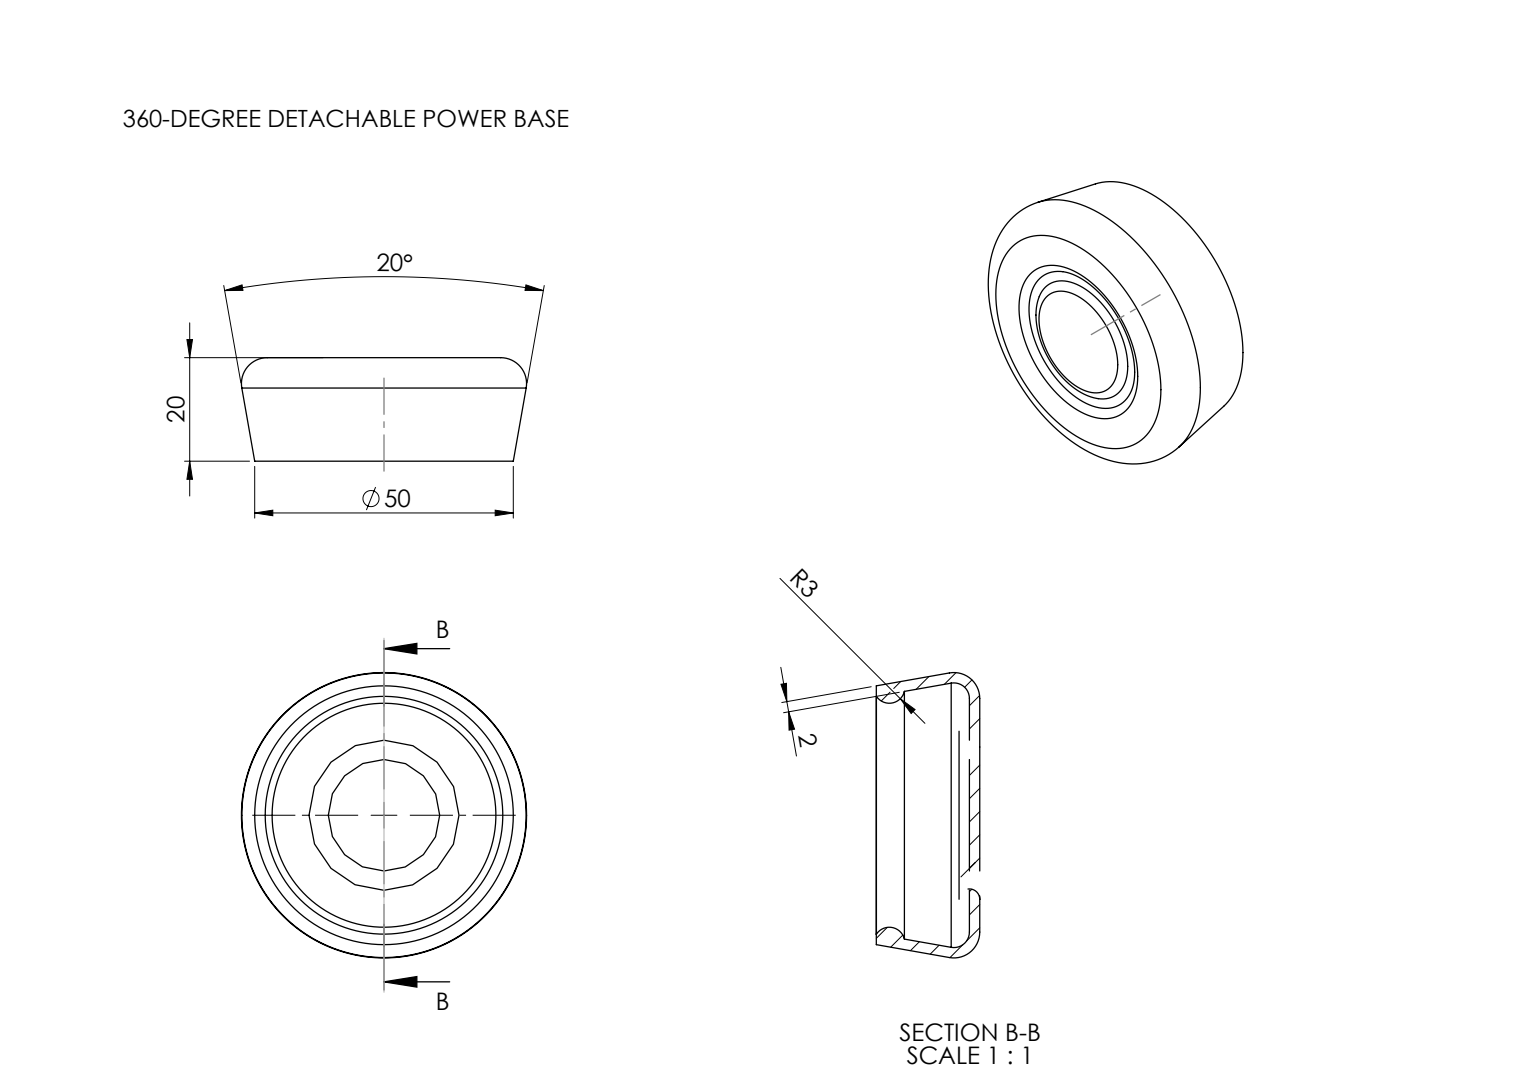
ISO-10303-21;
HEADER;
FILE_DESCRIPTION (('STEP AP214'),
    '1' );
FILE_NAME ('360-Degree Detachable Power Base.step',
    '2026-10-08T15:02:10',
    ( '' ),
    ( '' ),
    'SwSTEP 2.0',
    'SolidWorks 2026',
    '' );
FILE_SCHEMA (( 'AUTOMOTIVE_DESIGN' ));
ENDSEC;

DATA;
#9=ORIENTED_EDGE ( 'NONE', *, *, #11620, .F. ) ;
#88=AXIS2_PLACEMENT_3D ( 'NONE', #22054, #11930, #10248 ) ;
#91=AXIS2_PLACEMENT_3D ( 'NONE', #18121, #12939, #8104 ) ;
#101=CARTESIAN_POINT ( 'NONE',  ( -0.6349943332661909245, -10.75744069813302417, 92.00000000000001421 ) ) ;
#115=CARTESIAN_POINT ( 'NONE',  ( 23.92685091328690916, 0.000000000000000000, 80.43141006107198621 ) ) ;
#133=CIRCLE ( 'NONE', #6226, 27.49181041625929112 ) ;
#192=CIRCLE ( 'NONE', #12763, 23.92685091328691271 ) ;
#217=CARTESIAN_POINT ( 'NONE',  ( 0.000000000000000000, 0.000000000000000000, 75.00000000000000000 ) ) ;
#237=VERTEX_POINT ( 'NONE', #7603 ) ;
#250=EDGE_CURVE ( 'NONE', #10146, #1916, #14804, .T. ) ;
#282=SURFACE_STYLE_FILL_AREA ( #6812 ) ;
#298=ORIENTED_EDGE ( 'NONE', *, *, #2080, .T. ) ;
#311=DIRECTION ( 'NONE',  ( -0.1736481776669307198, 2.126576849575776229E-17, 0.9848077530122080203 ) ) ;
#428=ORIENTED_EDGE ( 'NONE', *, *, #5250, .F. ) ;
#434=DIRECTION ( 'NONE',  ( 0.000000000000000000, -1.000000000000000000, 0.000000000000000000 ) ) ;
#489=CARTESIAN_POINT ( 'NONE',  ( 0.000000000000000000, 0.000000000000000000, 75.01817430661621700 ) ) ;
#497=VERTEX_POINT ( 'NONE', #16816 ) ;
#506=CARTESIAN_POINT ( 'NONE',  ( 22.56777165119825668, 0.000000000000000000, 90.00000000000000000 ) ) ;
#515=LINE ( 'NONE', #19075, #11094 ) ;
#527=CARTESIAN_POINT ( 'NONE',  ( 0.000000000000000000, 0.000000000000000000, 93.00000000000000000 ) ) ;
#552=CARTESIAN_POINT ( 'NONE',  ( -10.76794919243112325, -2.704190363445815236E-15, 92.00000000000000000 ) ) ;
#572=LINE ( 'NONE', #18015, #14095 ) ;
#626=CARTESIAN_POINT ( 'NONE',  ( 0.000000000000000000, 0.000000000000000000, 94.00000000000000000 ) ) ;
#627=EDGE_CURVE ( 'NONE', #17378, #2791, #3286, .T. ) ;
#680=CARTESIAN_POINT ( 'NONE',  ( -1.701984465643862965, -14.42982486328545377, 93.00000000000000000 ) ) ;
#751=ADVANCED_FACE ( 'NONE', ( #21864, #18061 ), #2957, .F. ) ;
#779=CARTESIAN_POINT ( 'NONE',  ( 0.4310340159982882779, 14.49716617963122189, 93.00000000000001421 ) ) ;
#825=DIRECTION ( 'NONE',  ( 1.000000000000000000, 0.000000000000000000, 0.000000000000000000 ) ) ;
#840=DIRECTION ( 'NONE',  ( 1.000000000000000000, 0.000000000000000000, 0.000000000000000000 ) ) ;
#846=VERTEX_POINT ( 'NONE', #22098 ) ;
#895=CARTESIAN_POINT ( 'NONE',  ( -4.825543794723682112, 13.95218839875094829, 93.00000000000001421 ) ) ;
#912=CARTESIAN_POINT ( 'NONE',  ( 0.000000000000000000, 0.000000000000000000, 93.00000000000000000 ) ) ;
#930=VERTEX_POINT ( 'NONE', #1922 ) ;
#945=VERTEX_POINT ( 'NONE', #13560 ) ;
#980=CARTESIAN_POINT ( 'NONE',  ( 0.000000000000000000, 0.000000000000000000, 95.00000000000000000 ) ) ;
#1005=ORIENTED_EDGE ( 'NONE', *, *, #4139, .T. ) ;
#1007=CARTESIAN_POINT ( 'NONE',  ( 6.453512288987237611, 13.27786176931083695, 93.00000000000000000 ) ) ;
#1012=CARTESIAN_POINT ( 'NONE',  ( 13.08434944240164022, -7.394545551606342748, 92.99999999999998579 ) ) ;
#1024=DIRECTION ( 'NONE',  ( 1.000000000000000000, 0.000000000000000000, 0.000000000000000000 ) ) ;
#1027=EDGE_CURVE ( 'NONE', #7787, #237, #6904, .T. ) ;
#1132=DIRECTION ( 'NONE',  ( 1.000000000000000000, 0.000000000000000000, 0.000000000000000000 ) ) ;
#1155=AXIS2_PLACEMENT_3D ( 'NONE', #10454, #3681, #5262 ) ;
#1180=ORIENTED_EDGE ( 'NONE', *, *, #8054, .T. ) ;
#1188=AXIS2_PLACEMENT_3D ( 'NONE', #7802, #21501, #4395 ) ;
#1209=CONICAL_SURFACE ( 'NONE', #1910, 23.03038449397558196, 0.1745329251994333364 ) ;
#1245=CARTESIAN_POINT ( 'NONE',  ( 10.76794919243112325, 1.318693451189210089E-15, 93.00000000000000000 ) ) ;
#1307=VECTOR ( 'NONE', #17008, 1000.000000000000000 ) ;
#1311=ADVANCED_FACE ( 'NONE', ( #17464 ), #8333, .T. ) ;
#1322=FILL_AREA_STYLE_COLOUR ( '', #5562 ) ;
#1341=CARTESIAN_POINT ( 'NONE',  ( -14.49943138577569535, 0.2467007162552621036, 93.00000000000002842 ) ) ;
#1423=EDGE_CURVE ( 'NONE', #10960, #18642, #18111, .T. ) ;
#1436=EDGE_CURVE ( 'NONE', #1916, #930, #572, .T. ) ;
#1451=CARTESIAN_POINT ( 'NONE',  ( 10.76794919243112325, 0.000000000000000000, 92.00000000000000000 ) ) ;
#1464=CARTESIAN_POINT ( 'NONE',  ( 0.000000000000000000, 0.000000000000000000, 89.47905546699919910 ) ) ;
#1514=ORIENTED_EDGE ( 'NONE', *, *, #6789, .T. ) ;
#1566=CARTESIAN_POINT ( 'NONE',  ( 1.509788170712047295, -10.75822951548915007, 92.00000000000001421 ) ) ;
#1680=CARTESIAN_POINT ( 'NONE',  ( -7.838405800256100342, -7.387516090585425133, 92.00000000000000000 ) ) ;
#1686=ADVANCED_FACE ( 'NONE', ( #14531, #18010 ), #13270, .T. ) ;
#1755=CIRCLE ( 'NONE', #9316, 22.56777165119825668 ) ;
#1758=ORIENTED_EDGE ( 'NONE', *, *, #16835, .F. ) ;
#1790=CARTESIAN_POINT ( 'NONE',  ( 0.04718088033475073551, 10.76825293233556025, 91.99999999999998579 ) ) ;
#1832=EDGE_CURVE ( 'NONE', #18642, #10960, #2554, .T. ) ;
#1898=AXIS2_PLACEMENT_3D ( 'NONE', #489, #17488, #19159 ) ;
#1910=AXIS2_PLACEMENT_3D ( 'NONE', #9554, #18324, #18550 ) ;
#1916=VERTEX_POINT ( 'NONE', #20680 ) ;
#1922=CARTESIAN_POINT ( 'NONE',  ( -22.97235139684061878, 2.813301660702908866E-15, 75.01817430661621700 ) ) ;
#1975=CARTESIAN_POINT ( 'NONE',  ( -16.23205080756887853, 1.987852906508643644E-15, 93.00000000000000000 ) ) ;
#1976=EDGE_LOOP ( 'NONE', ( #12539, #12676 ) ) ;
#1979=DIRECTION ( 'NONE',  ( 1.000000000000000000, 0.000000000000000000, 0.000000000000000000 ) ) ;
#1982=CIRCLE ( 'NONE', #17819, 3.000000000000030198 ) ;
#1991=CARTESIAN_POINT ( 'NONE',  ( 0.000000000000000000, 0.000000000000000000, 89.47905546699919910 ) ) ;
#2000=ORIENTED_EDGE ( 'NONE', *, *, #16135, .T. ) ;
#2018=DIRECTION ( 'NONE',  ( 1.000000000000000000, 0.000000000000000000, 0.000000000000000000 ) ) ;
#2028=CIRCLE ( 'NONE', #16770, 23.92685091328691271 ) ;
#2068=ORIENTED_EDGE ( 'NONE', *, *, #1832, .F. ) ;
#2079=ORIENTED_EDGE ( 'NONE', *, *, #3880, .F. ) ;
#2080=EDGE_CURVE ( 'NONE', #10588, #846, #3065, .T. ) ;
#2089=DIRECTION ( 'NONE',  ( 1.000000000000000000, 0.000000000000000000, 0.000000000000000000 ) ) ;
#2124=CARTESIAN_POINT ( 'NONE',  ( -10.75744069813302417, 0.6349943332661998063, 92.00000000000000000 ) ) ;
#2128=DIRECTION ( 'NONE',  ( 0.000000000000000000, 0.000000000000000000, 1.000000000000000000 ) ) ;
#2143=CARTESIAN_POINT ( 'NONE',  ( 0.000000000000000000, 0.000000000000000000, 93.00000000000000000 ) ) ;
#2163=DIRECTION ( 'NONE',  ( 0.000000000000000000, 0.000000000000000000, 1.000000000000000000 ) ) ;
#2175=DIRECTION ( 'NONE',  ( 1.000000000000000000, 0.000000000000000000, 0.000000000000000000 ) ) ;
#2192=ADVANCED_FACE ( 'NONE', ( #8994 ), #7283, .T. ) ;
#2236=DIRECTION ( 'NONE',  ( 0.000000000000000000, 0.000000000000000000, -1.000000000000000000 ) ) ;
#2274=TOROIDAL_SURFACE ( 'NONE', #3700, 10.76794919243112325, 2.000000000000000000 ) ;
#2295=AXIS2_PLACEMENT_3D ( 'NONE', #9527, #19416, #4437 ) ;
#2358=EDGE_CURVE ( 'NONE', #20525, #20136, #5458, .T. ) ;
#2364=CIRCLE ( 'NONE', #7779, 25.52219491023488018 ) ;
#2425=DIRECTION ( 'NONE',  ( 0.000000000000000000, 0.000000000000000000, 1.000000000000000000 ) ) ;
#2452=AXIS2_PLACEMENT_3D ( 'NONE', #1975, #17738, #14032 ) ;
#2465=CARTESIAN_POINT ( 'NONE',  ( 10.60004861036625812, 9.899508790423018567, 93.00000000000001421 ) ) ;
#2554=B_SPLINE_CURVE_WITH_KNOTS ( 'NONE', 3,
 ( #16647, #17902, #11364, #9458, #4366, #21473, #2465, #9348, #9676, #16208, #1007, #13049, #19897, #20008, #779, #21811, #16319, #4485, #11470, #895, #5957, #18233, #12834, #7771, #16535, #7989, #6289, #13163, #4594, #18677, #3131, #10122, #6511, #1341, #15418, #15085, #16763 ),
 .UNSPECIFIED., .F., .F.,
 ( 4, 1, 1, 1, 1, 2, 2, 1, 1, 1, 1, 1, 2, 2, 1, 1, 1, 1, 1, 2, 2, 1, 1, 1, 1, 1, 2, 4 ),
 ( 0.000000000000000000, 0.06249999999999955591, 0.09374999999999931999, 0.1093749999999992090, 0.1171874999999991673, 0.1210937499999991673, 0.1249999999999991673, 0.1874999999999990008, 0.2187499999999988898, 0.2343749999999988343, 0.2421874999999988065, 0.2460937499999987788, 0.2480468749999987510, 0.2499999999999987788, 0.3124999999999985012, 0.3437499999999983902, 0.3593749999999983347, 0.3671874999999983347, 0.3710937499999982792, 0.3730468749999982792, 0.3749999999999982792, 0.4374999999999991118, 0.4687499999999995559, 0.4843749999999997780, 0.4921874999999998890, 0.4960937499999998890, 0.4980468749999999445, 0.5000000000000000000 ),
 .UNSPECIFIED. ) ;
#2582=AXIS2_PLACEMENT_3D ( 'NONE', #11523, #4313, #9844 ) ;
#2633=EDGE_CURVE ( 'NONE', #15441, #11225, #10382, .T. ) ;
#2661=VERTEX_POINT ( 'NONE', #13953 ) ;
#2665=AXIS2_PLACEMENT_3D ( 'NONE', #9411, #17753, #7839 ) ;
#2668=UNCERTAINTY_MEASURE_WITH_UNIT (LENGTH_MEASURE( 1.000000000000000082E-05 ), #5436, 'distance_accuracy_value', 'NONE');
#2693=CARTESIAN_POINT ( 'NONE',  ( -14.49031849020019003, -2.025093002184656488, 93.00000000000000000 ) ) ;
#2705=CARTESIAN_POINT ( 'NONE',  ( 0.000000000000000000, 0.000000000000000000, 93.00000000000000000 ) ) ;
#2707=DIRECTION ( 'NONE',  ( 1.000000000000000000, 0.000000000000000000, 0.000000000000000000 ) ) ;
#2791=VERTEX_POINT ( 'NONE', #12914 ) ;
#2814=DIRECTION ( 'NONE',  ( 0.000000000000000000, 0.000000000000000000, 1.000000000000000000 ) ) ;
#2837=CARTESIAN_POINT ( 'NONE',  ( -16.23205080756887853, 1.987852906508643644E-15, 95.00000000000000000 ) ) ;
#2853=VERTEX_POINT ( 'NONE', #17880 ) ;
#2888=AXIS2_PLACEMENT_3D ( 'NONE', #4214, #14918, #840 ) ;
#2957=PLANE ( 'NONE',  #2582 ) ;
#3012=ORIENTED_EDGE ( 'NONE', *, *, #250, .T. ) ;
#3015=CARTESIAN_POINT ( 'NONE',  ( 7.354678144329572120, -7.869443266638024070, 92.00000000000000000 ) ) ;
#3026=CARTESIAN_POINT ( 'NONE',  ( 8.476473295508071715, 6.680697330908218490, 92.00000000000002842 ) ) ;
#3065=B_SPLINE_CURVE_WITH_KNOTS ( 'NONE', 3,
 ( #13724, #12032, #22158, #15194, #11810, #4820, #1680, #9899, #6856, #18784, #6971, #16987, #20338, #17208, #101, #15518, #8324, #13843, #11918, #1566, #11697, #8554, #6747, #11577, #3015, #4934, #18566, #8441, #10011, #1451 ),
 .UNSPECIFIED., .F., .F.,
 ( 4, 1, 1, 1, 1, 1, 2, 2, 1, 1, 1, 1, 1, 2, 2, 1, 1, 1, 1, 2, 2, 4 ),
 ( 0.5000000000000000000, 0.5625000000000000000, 0.5937500000000000000, 0.6093750000000001110, 0.6171875000000001110, 0.6210937500000001110, 0.6230468750000001110, 0.6250000000000001110, 0.6875000000000002220, 0.7187500000000003331, 0.7343750000000003331, 0.7421875000000003331, 0.7460937500000003331, 0.7480468750000003331, 0.7500000000000004441, 0.8125000000000004441, 0.8437500000000004441, 0.8593750000000005551, 0.8671875000000005551, 0.8710937500000006661, 0.8750000000000006661, 1.000000000000000000 ),
 .UNSPECIFIED. ) ;
#3073=EDGE_CURVE ( 'NONE', #2853, #20136, #1755, .T. ) ;
#3111=( LENGTH_UNIT ( ) NAMED_UNIT ( * ) SI_UNIT ( .MILLI., .METRE. ) );
#3131=CARTESIAN_POINT ( 'NONE',  ( -14.42982486328545200, 1.701984465643896272, 93.00000000000001421 ) ) ;
#3140=CARTESIAN_POINT ( 'NONE',  ( 0.3188271712753663611, 10.76635261883074257, 92.00000000000001421 ) ) ;
#3142=FACE_BOUND ( 'NONE', #22130, .T. ) ;
#3168=AXIS2_PLACEMENT_3D ( 'NONE', #13351, #18422, #4789 ) ;
#3286=CIRCLE ( 'NONE', #10846, 10.76794919243112325 ) ;
#3316=AXIS2_PLACEMENT_3D ( 'NONE', #1464, #11824, #18690 ) ;
#3322=ORIENTED_EDGE ( 'NONE', *, *, #12216, .F. ) ;
#3334=DIRECTION ( 'NONE',  ( 1.224646799147353207E-16, 1.000000000000000000, -0.000000000000000000 ) ) ;
#3348=ORIENTED_EDGE ( 'NONE', *, *, #13732, .T. ) ;
#3361=EDGE_CURVE ( 'NONE', #6741, #945, #20046, .T. ) ;
#3465=ORIENTED_EDGE ( 'NONE', *, *, #250, .F. ) ;
#3530=SURFACE_STYLE_USAGE ( .BOTH. , #18954 ) ;
#3630=EDGE_CURVE ( 'NONE', #4483, #16572, #12535, .T. ) ;
#3633=ORIENTED_EDGE ( 'NONE', *, *, #20686, .F. ) ;
#3681=DIRECTION ( 'NONE',  ( -0.000000000000000000, -0.000000000000000000, 1.000000000000000000 ) ) ;
#3688=AXIS2_PLACEMENT_3D ( 'NONE', #12548, #7157, #12442 ) ;
#3700=AXIS2_PLACEMENT_3D ( 'NONE', #20546, #10329, #10549 ) ;
#3795=CIRCLE ( 'NONE', #21027, 2.000000000000001776 ) ;
#3806=B_SPLINE_CURVE_WITH_KNOTS ( 'NONE', 3,
 ( #6756, #8666, #5160, #4944, #3026, #8563, #18578, #20235, #10023, #20123, #4831, #11928, #15427, #6865, #3140, #11590, #15529, #1790, #18462, #9913, #16776, #8224, #6522, #13392, #8335, #11820, #12378, #3809, #17662, #19008, #17325, #2124, #17779, #10462, #8895, #13961, #552 ),
 .UNSPECIFIED., .F., .F.,
 ( 4, 1, 1, 1, 1, 2, 2, 1, 1, 1, 1, 1, 2, 2, 1, 1, 1, 1, 1, 2, 2, 1, 1, 1, 1, 1, 2, 4 ),
 ( 0.000000000000000000, 0.06250000000000048572, 0.09375000000000069389, 0.1093750000000008049, 0.1171875000000008604, 0.1210937500000009159, 0.1250000000000009714, 0.1875000000000012212, 0.2187500000000013600, 0.2343750000000014433, 0.2421875000000014710, 0.2460937500000014710, 0.2480468750000014710, 0.2500000000000014988, 0.3125000000000016653, 0.3437500000000017208, 0.3593750000000017764, 0.3671875000000017764, 0.3710937500000017764, 0.3730468750000017208, 0.3750000000000016653, 0.4375000000000008882, 0.4687500000000004996, 0.4843750000000002776, 0.4921875000000001665, 0.4960937500000000555, 0.4980468750000000555, 0.5000000000000000000 ),
 .UNSPECIFIED. ) ;
#3809=CARTESIAN_POINT ( 'NONE',  ( -8.674798497629360838, 6.539635590297948831, 91.99999999999997158 ) ) ;
#3822=AXIS2_PLACEMENT_3D ( 'NONE', #18252, #2814, #13071 ) ;
#3880=EDGE_CURVE ( 'NONE', #10146, #945, #515, .T. ) ;
#3886=SHAPE_REPRESENTATION_RELATIONSHIP ( 'NONE' , 'NONE' ,  #8462, #21175 ) ;
#3889=ORIENTED_EDGE ( 'NONE', *, *, #8253, .F. ) ;
#3912=ORIENTED_EDGE ( 'NONE', *, *, #3073, .F. ) ;
#3931=ORIENTED_EDGE ( 'NONE', *, *, #17519, .T. ) ;
#3969=ORIENTED_EDGE ( 'NONE', *, *, #8054, .F. ) ;
#4000=FACE_OUTER_BOUND ( 'NONE', #15773, .T. ) ;
#4003=EDGE_CURVE ( 'NONE', #12254, #20879, #20779, .T. ) ;
#4023=UNCERTAINTY_MEASURE_WITH_UNIT (LENGTH_MEASURE( 1.000000000000000082E-05 ), #4912, 'distance_accuracy_value', 'NONE');
#4042=TOROIDAL_SURFACE ( 'NONE', #8734, 22.56777165119825668, 5.000000000000000000 ) ;
#4049=CARTESIAN_POINT ( 'NONE',  ( -0.06328415631827169485, -14.50030254718124390, 92.99999999999998579 ) ) ;
#4084=FACE_OUTER_BOUND ( 'NONE', #17806, .T. ) ;
#4093=TOROIDAL_SURFACE ( 'NONE', #2665, 24.63401512838761320, 3.000000000000035083 ) ;
#4139=EDGE_CURVE ( 'NONE', #21337, #16572, #10736, .T. ) ;
#4160=CARTESIAN_POINT ( 'NONE',  ( 14.50000000000000000, 0.000000000000000000, 93.00000000000000000 ) ) ;
#4169=ADVANCED_FACE ( 'NONE', ( #20868 ), #14696, .T. ) ;
#4170=EDGE_LOOP ( 'NONE', ( #21486, #15699, #13268, #3912 ) ) ;
#4194=DIRECTION ( 'NONE',  ( -1.000000000000000000, -1.224646799147353454E-16, 0.000000000000000000 ) ) ;
#4214=CARTESIAN_POINT ( 'NONE',  ( 0.000000000000000000, 0.000000000000000000, 75.34729635533385306 ) ) ;
#4269=CARTESIAN_POINT ( 'NONE',  ( -14.50000000000000000, 1.775737858763662015E-15, 93.00000000000000000 ) ) ;
#4313=DIRECTION ( 'NONE',  ( 0.000000000000000000, 0.000000000000000000, 1.000000000000000000 ) ) ;
#4357=DIRECTION ( 'NONE',  ( -0.000000000000000000, -0.000000000000000000, -1.000000000000000000 ) ) ;
#4366=CARTESIAN_POINT ( 'NONE',  ( 11.41432417523484055, 8.992600385930652251, 93.00000000000000000 ) ) ;
#4372=CARTESIAN_POINT ( 'NONE',  ( -10.42709000561872834, -10.07820250684338603, 93.00000000000001421 ) ) ;
#4380=ORIENTED_EDGE ( 'NONE', *, *, #12449, .F. ) ;
#4395=DIRECTION ( 'NONE',  ( 1.000000000000000000, 0.000000000000000000, 0.000000000000000000 ) ) ;
#4437=DIRECTION ( 'NONE',  ( 1.000000000000000000, 0.000000000000000000, 0.000000000000000000 ) ) ;
#4445=DIRECTION ( 'NONE',  ( 0.000000000000000000, -1.000000000000000000, 0.000000000000000000 ) ) ;
#4483=VERTEX_POINT ( 'NONE', #18176 ) ;
#4485=CARTESIAN_POINT ( 'NONE',  ( 0.06328415631827062626, 14.50030254718124212, 92.99999999999997158 ) ) ;
#4579=CARTESIAN_POINT ( 'NONE',  ( 0.000000000000000000, 0.000000000000000000, 89.13175911166534604 ) ) ;
#4594=CARTESIAN_POINT ( 'NONE',  ( -13.27786176931083162, 6.453512288987280243, 92.99999999999998579 ) ) ;
#4657=ORIENTED_EDGE ( 'NONE', *, *, #13403, .T. ) ;
#4776=AXIS2_PLACEMENT_3D ( 'NONE', #12920, #16411, #9331 ) ;
#4789=DIRECTION ( 'NONE',  ( 1.000000000000000000, 0.000000000000000000, 0.000000000000000000 ) ) ;
#4790=ORIENTED_EDGE ( 'NONE', *, *, #20520, .F. ) ;
#4820=CARTESIAN_POINT ( 'NONE',  ( -8.055668064929562888, -7.157650466794454935, 91.99999999999997158 ) ) ;
#4831=CARTESIAN_POINT ( 'NONE',  ( 4.782033626261160464, 9.864562363145058299, 92.00000000000000000 ) ) ;
#4912=( LENGTH_UNIT ( ) NAMED_UNIT ( * ) SI_UNIT ( .MILLI., .METRE. ) );
#4934=CARTESIAN_POINT ( 'NONE',  ( 7.485089409085513346, -7.743278074783935594, 91.99999999999998579 ) ) ;
#4944=CARTESIAN_POINT ( 'NONE',  ( 9.223872243966841467, 5.696734612111038487, 92.00000000000001421 ) ) ;
#4951=DIRECTION ( 'NONE',  ( -0.000000000000000000, -0.000000000000000000, 1.000000000000000000 ) ) ;
#5042=ORIENTED_EDGE ( 'NONE', *, *, #13039, .F. ) ;
#5059=DIRECTION ( 'NONE',  ( 1.000000000000000000, 0.000000000000000000, 0.000000000000000000 ) ) ;
#5077=ORIENTED_EDGE ( 'NONE', *, *, #1027, .F. ) ;
#5101=EDGE_LOOP ( 'NONE', ( #14716, #20263, #18999, #19285 ) ) ;
#5132=CIRCLE ( 'NONE', #10175, 25.00000000000000000 ) ;
#5160=CARTESIAN_POINT ( 'NONE',  ( 10.37371678005726139, 3.577098705721246219, 91.99999999999998579 ) ) ;
#5216=ORIENTED_EDGE ( 'NONE', *, *, #21646, .F. ) ;
#5250=EDGE_CURVE ( 'NONE', #21337, #12667, #10141, .T. ) ;
#5262=DIRECTION ( 'NONE',  ( 1.000000000000000000, 0.000000000000000000, 0.000000000000000000 ) ) ;
#5317=AXIS2_PLACEMENT_3D ( 'NONE', #11889, #6371, #14944 ) ;
#5323=ORIENTED_EDGE ( 'NONE', *, *, #3630, .F. ) ;
#5332=DIRECTION ( 'NONE',  ( 0.000000000000000000, 0.000000000000000000, 1.000000000000000000 ) ) ;
#5387=ORIENTED_EDGE ( 'NONE', *, *, #10065, .T. ) ;
#5436=( LENGTH_UNIT ( ) NAMED_UNIT ( * ) SI_UNIT ( .MILLI., .METRE. ) );
#5443=CARTESIAN_POINT ( 'NONE',  ( 0.000000000000000000, 0.000000000000000000, 77.51594804401857175 ) ) ;
#5458=CIRCLE ( 'NONE', #12440, 5.000000000000004441 ) ;
#5465=VERTEX_POINT ( 'NONE', #15166 ) ;
#5494=AXIS2_PLACEMENT_3D ( 'NONE', #5443, #5670, #19502 ) ;
#5518=DIRECTION ( 'NONE',  ( -1.000000000000000000, 1.224646799147353454E-16, 0.000000000000000000 ) ) ;
#5562=COLOUR_RGB ( '', 0.40784314, 0.44705882, 0.49803922) ;
#5670=DIRECTION ( 'NONE',  ( -0.000000000000000000, -0.000000000000000000, 1.000000000000000000 ) ) ;
#5698=ADVANCED_FACE ( 'NONE', ( #21204 ), #5824, .F. ) ;
#5722=CARTESIAN_POINT ( 'NONE',  ( 0.000000000000000000, 0.000000000000000000, 93.00000000000000000 ) ) ;
#5736=CARTESIAN_POINT ( 'NONE',  ( -3.344898002356346378, -14.20274344593240912, 93.00000000000001421 ) ) ;
#5802=DIRECTION ( 'NONE',  ( 1.000000000000000000, 0.000000000000000000, 0.000000000000000000 ) ) ;
#5824=TOROIDAL_SURFACE ( 'NONE', #7991, 22.56777165119825668, 3.000000000000000000 ) ;
#5825=EDGE_CURVE ( 'NONE', #20879, #12254, #6862, .T. ) ;
#5830=CARTESIAN_POINT ( 'NONE',  ( 0.000000000000000000, 0.000000000000000000, 75.01817430661621700 ) ) ;
#5847=CARTESIAN_POINT ( 'NONE',  ( -0.2467007162552578292, -14.49943138577569357, 93.00000000000002842 ) ) ;
#5883=DIRECTION ( 'NONE',  ( -1.224646799147353207E-16, 1.000000000000000000, 0.000000000000000000 ) ) ;
#5902=DIRECTION ( 'NONE',  ( 0.000000000000000000, 0.000000000000000000, 1.000000000000000000 ) ) ;
#5939=ADVANCED_FACE ( 'NONE', ( #19305 ), #14769, .F. ) ;
#5942=LINE ( 'NONE', #13149, #19177 ) ;
#5944=VECTOR ( 'NONE', #311, 1000.000000000000000 ) ;
#5955=ORIENTED_EDGE ( 'NONE', *, *, #3361, .F. ) ;
#5957=CARTESIAN_POINT ( 'NONE',  ( -7.677656142228050484, 12.40805626191516353, 93.00000000000000000 ) ) ;
#5986=DIRECTION ( 'NONE',  ( 1.000000000000000000, 0.000000000000000000, -0.000000000000000000 ) ) ;
#6011=CARTESIAN_POINT ( 'NONE',  ( 0.000000000000000000, 0.000000000000000000, 95.00000000000000000 ) ) ;
#6020=ORIENTED_EDGE ( 'NONE', *, *, #18896, .F. ) ;
#6108=DIRECTION ( 'NONE',  ( 0.000000000000000000, 0.000000000000000000, 1.000000000000000000 ) ) ;
#6137=ORIENTED_EDGE ( 'NONE', *, *, #7781, .T. ) ;
#6179=CARTESIAN_POINT ( 'NONE',  ( 10.07835692657692128, -10.42743089613093233, 93.00000000000002842 ) ) ;
#6193=CARTESIAN_POINT ( 'NONE',  ( -23.92685091328690916, 2.930194138463273749E-15, 80.43141006107198621 ) ) ;
#6226=AXIS2_PLACEMENT_3D ( 'NONE', #4579, #6381, #11234 ) ;
#6230=ADVANCED_FACE ( 'NONE', ( #7830 ), #12616, .F. ) ;
#6233=DIRECTION ( 'NONE',  ( 1.000000000000000000, 0.000000000000000000, 0.000000000000000000 ) ) ;
#6267=CIRCLE ( 'NONE', #14209, 2.000000000000000000 ) ;
#6280=DIRECTION ( 'NONE',  ( -1.000000000000000000, 0.000000000000000000, 0.000000000000000000 ) ) ;
#6289=CARTESIAN_POINT ( 'NONE',  ( -10.20851360429410981, 10.29801091644274180, 92.99999999999998579 ) ) ;
#6298=CIRCLE ( 'NONE', #16361, 3.000000000000002665 ) ;
#6309=DIRECTION ( 'NONE',  ( 0.000000000000000000, 0.000000000000000000, 1.000000000000000000 ) ) ;
#6334=CARTESIAN_POINT ( 'NONE',  ( 0.000000000000000000, 0.000000000000000000, 75.00000000000000000 ) ) ;
#6371=DIRECTION ( 'NONE',  ( 0.000000000000000000, -1.000000000000000000, 0.000000000000000000 ) ) ;
#6381=DIRECTION ( 'NONE',  ( -0.000000000000000000, -0.000000000000000000, -1.000000000000000000 ) ) ;
#6397=ORIENTED_EDGE ( 'NONE', *, *, #3880, .T. ) ;
#6477=ORIENTED_EDGE ( 'NONE', *, *, #1436, .F. ) ;
#6511=CARTESIAN_POINT ( 'NONE',  ( -14.49716617963121834, 0.4310340159982911645, 92.99999999999997158 ) ) ;
#6522=CARTESIAN_POINT ( 'NONE',  ( -7.157650466794449606, 8.055668064929562888, 92.00000000000001421 ) ) ;
#6582=DIRECTION ( 'NONE',  ( -0.000000000000000000, -0.000000000000000000, 1.000000000000000000 ) ) ;
#6677=AXIS2_PLACEMENT_3D ( 'NONE', #18028, #16226, #2707 ) ;
#6741=VERTEX_POINT ( 'NONE', #16173 ) ;
#6747=CARTESIAN_POINT ( 'NONE',  ( 6.688043756404092655, -8.469031667849375111, 92.00000000000000000 ) ) ;
#6756=CARTESIAN_POINT ( 'NONE',  ( 10.76794919243112325, 0.000000000000000000, 92.00000000000000000 ) ) ;
#6789=EDGE_CURVE ( 'NONE', #497, #10628, #2364, .T. ) ;
#6812=FILL_AREA_STYLE ('',( #12099 ) ) ;
#6829=ORIENTED_EDGE ( 'NONE', *, *, #5250, .T. ) ;
#6856=CARTESIAN_POINT ( 'NONE',  ( -7.678935899902896267, -7.549707216296320134, 92.00000000000001421 ) ) ;
#6862=CIRCLE ( 'NONE', #7937, 12.50000000000000000 ) ;
#6865=CARTESIAN_POINT ( 'NONE',  ( 0.6349943332661940332, 10.75744069813302595, 92.00000000000002842 ) ) ;
#6878=ORIENTED_EDGE ( 'NONE', *, *, #14385, .F. ) ;
#6904=CIRCLE ( 'NONE', #19462, 3.000000000000033751 ) ;
#6923=PRESENTATION_STYLE_ASSIGNMENT (( #3530 ) ) ;
#6940=CARTESIAN_POINT ( 'NONE',  ( 0.000000000000000000, 0.000000000000000000, 94.00000000000000000 ) ) ;
#6971=CARTESIAN_POINT ( 'NONE',  ( -6.539635590297925738, -8.674798497629369720, 92.00000000000001421 ) ) ;
#7000=STYLED_ITEM ( 'NONE', ( #6923 ), #14295 ) ;
#7020=( GEOMETRIC_REPRESENTATION_CONTEXT ( 3 ) GLOBAL_UNCERTAINTY_ASSIGNED_CONTEXT ( ( #4023 ) ) GLOBAL_UNIT_ASSIGNED_CONTEXT ( ( #4912, #11897, #17080 ) ) REPRESENTATION_CONTEXT ( 'NONE', 'WORKASPACE' ) );
#7060=CARTESIAN_POINT ( 'NONE',  ( 0.000000000000000000, 0.000000000000000000, 90.00000000000000000 ) ) ;
#7067=DIRECTION ( 'NONE',  ( 1.000000000000000000, 0.000000000000000000, 0.000000000000000000 ) ) ;
#7071=AXIS2_PLACEMENT_3D ( 'NONE', #912, #6309, #1132 ) ;
#7086=DIRECTION ( 'NONE',  ( 1.000000000000000000, 0.000000000000000000, 0.000000000000000000 ) ) ;
#7107=EDGE_LOOP ( 'NONE', ( #20848, #8716 ) ) ;
#7157=DIRECTION ( 'NONE',  ( 0.000000000000000000, 0.000000000000000000, 1.000000000000000000 ) ) ;
#7192=ORIENTED_EDGE ( 'NONE', *, *, #3073, .T. ) ;
#7218=ORIENTED_EDGE ( 'NONE', *, *, #20925, .F. ) ;
#7259=ORIENTED_EDGE ( 'NONE', *, *, #627, .T. ) ;
#7272=ORIENTED_EDGE ( 'NONE', *, *, #21646, .T. ) ;
#7283=TOROIDAL_SURFACE ( 'NONE', #1155, 24.63401512838761320, 3.000000000000035083 ) ;
#7292=LINE ( 'NONE', #15734, #5944 ) ;
#7382=DIRECTION ( 'NONE',  ( 0.000000000000000000, 0.000000000000000000, -1.000000000000000000 ) ) ;
#7391=DIRECTION ( 'NONE',  ( 1.000000000000000000, 0.000000000000000000, 0.000000000000000000 ) ) ;
#7413=ORIENTED_EDGE ( 'NONE', *, *, #12216, .T. ) ;
#7448=CARTESIAN_POINT ( 'NONE',  ( 4.825543794723634150, -13.95218839875094119, 92.99999999999997158 ) ) ;
#7481=ORIENTED_EDGE ( 'NONE', *, *, #6789, .F. ) ;
#7496=EDGE_CURVE ( 'NONE', #14323, #2661, #14623, .T. ) ;
#7502=DIRECTION ( 'NONE',  ( 0.000000000000000000, 0.000000000000000000, 1.000000000000000000 ) ) ;
#7546=EDGE_CURVE ( 'NONE', #16572, #4483, #16413, .T. ) ;
#7554=CARTESIAN_POINT ( 'NONE',  ( -13.95218839875094119, -4.825543794723769153, 93.00000000000000000 ) ) ;
#7591=DIRECTION ( 'NONE',  ( 0.000000000000000000, 0.000000000000000000, -1.000000000000000000 ) ) ;
#7603=CARTESIAN_POINT ( 'NONE',  ( -21.63401512838757768, 2.649402737968526106E-15, 77.51594804401857175 ) ) ;
#7661=VECTOR ( 'NONE', #14357, 1000.000000000000000 ) ;
#7732=EDGE_CURVE ( 'NONE', #237, #930, #22164, .T. ) ;
#7771=CARTESIAN_POINT ( 'NONE',  ( -9.946257437971052440, 10.55583158923998077, 93.00000000000001421 ) ) ;
#7779=AXIS2_PLACEMENT_3D ( 'NONE', #1991, #12356, #5802 ) ;
#7781=EDGE_CURVE ( 'NONE', #2661, #14323, #7792, .T. ) ;
#7787=VERTEX_POINT ( 'NONE', #6193 ) ;
#7792=CIRCLE ( 'NONE', #14977, 22.56777165119825668 ) ;
#7802=CARTESIAN_POINT ( 'NONE',  ( 0.000000000000000000, 0.000000000000000000, 89.13175911166534604 ) ) ;
#7830=FACE_OUTER_BOUND ( 'NONE', #16877, .T. ) ;
#7839=DIRECTION ( 'NONE',  ( 1.000000000000000000, 0.000000000000000000, 0.000000000000000000 ) ) ;
#7855=DIRECTION ( 'NONE',  ( 0.000000000000000000, 0.000000000000000000, 1.000000000000000000 ) ) ;
#7873=CARTESIAN_POINT ( 'NONE',  ( 0.000000000000000000, 0.000000000000000000, 93.00000000000000000 ) ) ;
#7887=CARTESIAN_POINT ( 'NONE',  ( -10.84906991693323164, -9.635142796197690984, 93.00000000000001421 ) ) ;
#7937=AXIS2_PLACEMENT_3D ( 'NONE', #626, #10656, #2089 ) ;
#7962=ORIENTED_EDGE ( 'NONE', *, *, #5825, .T. ) ;
#7987=EDGE_LOOP ( 'NONE', ( #428, #1005, #5323, #17175 ) ) ;
#7989=CARTESIAN_POINT ( 'NONE',  ( -10.16585704662448641, 10.34058050218014557, 93.00000000000000000 ) ) ;
#7991=AXIS2_PLACEMENT_3D ( 'NONE', #7060, #7502, #1979 ) ;
#8043=AXIS2_PLACEMENT_3D ( 'NONE', #17298, #3334, #10216 ) ;
#8054=EDGE_CURVE ( 'NONE', #11225, #20525, #14054, .T. ) ;
#8104=DIRECTION ( 'NONE',  ( 1.000000000000000000, 0.000000000000000000, -0.000000000000000000 ) ) ;
#8192=CARTESIAN_POINT ( 'NONE',  ( 25.00000000000000000, 0.000000000000000000, 75.00000000000000000 ) ) ;
#8224=CARTESIAN_POINT ( 'NONE',  ( -6.688043756404080220, 8.469031667849378664, 92.00000000000001421 ) ) ;
#8244=CARTESIAN_POINT ( 'NONE',  ( 0.000000000000000000, 0.000000000000000000, 95.00000000000000000 ) ) ;
#8253=EDGE_CURVE ( 'NONE', #15223, #7787, #2028, .T. ) ;
#8289=ORIENTED_EDGE ( 'NONE', *, *, #15957, .F. ) ;
#8324=CARTESIAN_POINT ( 'NONE',  ( -0.1824719560092676052, -10.76782065184847959, 92.00000000000002842 ) ) ;
#8333=TOROIDAL_SURFACE ( 'NONE', #20898, 16.23205080756887853, 2.000000000000000000 ) ;
#8335=CARTESIAN_POINT ( 'NONE',  ( -7.484971844052076939, 7.743026158993130181, 91.99999999999998579 ) ) ;
#8339=PRODUCT_DEFINITION_SHAPE ( 'NONE', 'NONE',  #17443 ) ;
#8364=CIRCLE ( 'NONE', #3316, 25.52219491023488018 ) ;
#8441=CARTESIAN_POINT ( 'NONE',  ( 9.716662759434166574, -5.484269832949179246, 92.00000000000002842 ) ) ;
#8462=SHAPE_REPRESENTATION ( '360-Degree Detachable Power Base', ( #6677 ), #10247 ) ;
#8554=CARTESIAN_POINT ( 'NONE',  ( 5.709328484389686764, -9.211115167980509000, 91.99999999999998579 ) ) ;
#8563=CARTESIAN_POINT ( 'NONE',  ( 8.059654651175295115, 7.153714881707382567, 92.00000000000001421 ) ) ;
#8576=ORIENTED_EDGE ( 'NONE', *, *, #1423, .F. ) ;
#8642=FACE_OUTER_BOUND ( 'NONE', #16446, .T. ) ;
#8666=CARTESIAN_POINT ( 'NONE',  ( 10.76794919243112680, 1.500192839452123339, 91.99999999999997158 ) ) ;
#8706=AXIS2_PLACEMENT_3D ( 'NONE', #9191, #10763, #17628 ) ;
#8716=ORIENTED_EDGE ( 'NONE', *, *, #2633, .F. ) ;
#8734=AXIS2_PLACEMENT_3D ( 'NONE', #10949, #19378, #16020 ) ;
#8790=DIRECTION ( 'NONE',  ( 0.000000000000000000, 0.000000000000000000, 1.000000000000000000 ) ) ;
#8845=CARTESIAN_POINT ( 'NONE',  ( 22.56777165119825668, 0.000000000000000000, 95.00000000000000000 ) ) ;
#8895=CARTESIAN_POINT ( 'NONE',  ( -10.76827681573429984, 0.09137847850202132638, 92.00000000000000000 ) ) ;
#8907=ORIENTED_EDGE ( 'NONE', *, *, #4003, .F. ) ;
#8913=DIRECTION ( 'NONE',  ( 1.000000000000000000, 0.000000000000000000, 0.000000000000000000 ) ) ;
#8948=EDGE_LOOP ( 'NONE', ( #12915, #10235, #13161, #15879 ) ) ;
#8982=EDGE_CURVE ( 'NONE', #12667, #4483, #12329, .T. ) ;
#8983=FACE_OUTER_BOUND ( 'NONE', #22238, .T. ) ;
#8994=FACE_OUTER_BOUND ( 'NONE', #13948, .T. ) ;
#9043=DIRECTION ( 'NONE',  ( 1.000000000000000000, 0.000000000000000000, 0.000000000000000000 ) ) ;
#9090=AXIS2_PLACEMENT_3D ( 'NONE', #5722, #8790, #9117 ) ;
#9102=CARTESIAN_POINT ( 'NONE',  ( 22.56777165119825668, 0.000000000000000000, 90.00000000000000000 ) ) ;
#9117=DIRECTION ( 'NONE',  ( 1.000000000000000000, 0.000000000000000000, 0.000000000000000000 ) ) ;
#9191=CARTESIAN_POINT ( 'NONE',  ( 0.000000000000000000, 0.000000000000000000, 75.34729635533385306 ) ) ;
#9219=ORIENTED_EDGE ( 'NONE', *, *, #2358, .F. ) ;
#9247=CARTESIAN_POINT ( 'NONE',  ( 7.677656142228014957, -12.40805626191516353, 93.00000000000000000 ) ) ;
#9279=CARTESIAN_POINT ( 'NONE',  ( 0.000000000000000000, 0.000000000000000000, 90.00000000000000000 ) ) ;
#9289=ORIENTED_EDGE ( 'NONE', *, *, #1436, .T. ) ;
#9300=ADVANCED_FACE ( 'NONE', ( #11061 ), #4042, .T. ) ;
#9316=AXIS2_PLACEMENT_3D ( 'NONE', #980, #7855, #21557 ) ;
#9326=ORIENTED_EDGE ( 'NONE', *, *, #9377, .T. ) ;
#9331=DIRECTION ( 'NONE',  ( 1.000000000000000000, 0.000000000000000000, 0.000000000000000000 ) ) ;
#9348=CARTESIAN_POINT ( 'NONE',  ( 10.42862217565707894, 10.07717698332843170, 92.99999999999998579 ) ) ;
#9377=EDGE_CURVE ( 'NONE', #930, #945, #20937, .T. ) ;
#9407=ORIENTED_EDGE ( 'NONE', *, *, #5825, .F. ) ;
#9411=CARTESIAN_POINT ( 'NONE',  ( 0.000000000000000000, 0.000000000000000000, 77.51594804401857175 ) ) ;
#9458=CARTESIAN_POINT ( 'NONE',  ( 12.42076324352741956, 7.665070080910708405, 93.00000000000000000 ) ) ;
#9464=CARTESIAN_POINT ( 'NONE',  ( 2.025093002184578772, -14.49031849020018470, 93.00000000000000000 ) ) ;
#9518=SHAPE_DEFINITION_REPRESENTATION ( #8339, #8462 ) ;
#9527=CARTESIAN_POINT ( 'NONE',  ( 0.000000000000000000, 0.000000000000000000, 95.00000000000000000 ) ) ;
#9554=CARTESIAN_POINT ( 'NONE',  ( 0.000000000000000000, 0.000000000000000000, 75.34729635533385306 ) ) ;
#9575=CARTESIAN_POINT ( 'NONE',  ( 9.635142796197660786, -10.84906991693322453, 93.00000000000001421 ) ) ;
#9589=DIRECTION ( 'NONE',  ( 0.000000000000000000, 0.000000000000000000, 1.000000000000000000 ) ) ;
#9600=ADVANCED_FACE ( 'NONE', ( #14337 ), #19508, .F. ) ;
#9663=DIRECTION ( 'NONE',  ( 0.000000000000000000, 0.000000000000000000, 1.000000000000000000 ) ) ;
#9667=FACE_OUTER_BOUND ( 'NONE', #21194, .T. ) ;
#9676=CARTESIAN_POINT ( 'NONE',  ( 10.34297350568055052, 10.16397888138328121, 93.00000000000001421 ) ) ;
#9693=CARTESIAN_POINT ( 'NONE',  ( -24.63401512838761320, 3.016796777712736283E-15, 77.51594804401857175 ) ) ;
#9735=ADVANCED_FACE ( 'NONE', ( #19704 ), #16678, .T. ) ;
#9818=AXIS2_PLACEMENT_3D ( 'NONE', #8244, #11609, #5986 ) ;
#9844=DIRECTION ( 'NONE',  ( 1.000000000000000000, 0.000000000000000000, -0.000000000000000000 ) ) ;
#9855=AXIS2_PLACEMENT_3D ( 'NONE', #21878, #6582, #9969 ) ;
#9899=CARTESIAN_POINT ( 'NONE',  ( -7.743026158993134622, -7.484971844052081380, 92.00000000000000000 ) ) ;
#9913=CARTESIAN_POINT ( 'NONE',  ( -3.593890535426079946, 10.35670734540881455, 92.00000000000001421 ) ) ;
#9969=DIRECTION ( 'NONE',  ( 1.000000000000000000, 0.000000000000000000, 0.000000000000000000 ) ) ;
#10011=CARTESIAN_POINT ( 'NONE',  ( 10.76794919243112680, -2.946239868469075596, 92.00000000000000000 ) ) ;
#10023=CARTESIAN_POINT ( 'NONE',  ( 7.681243287386652518, 7.547795605678436104, 91.99999999999998579 ) ) ;
#10065=EDGE_CURVE ( 'NONE', #20525, #5465, #17023, .T. ) ;
#10101=PRESENTATION_STYLE_ASSIGNMENT (( #22013 ) ) ;
#10122=CARTESIAN_POINT ( 'NONE',  ( -14.48452571672253342, 0.8583760989383736328, 93.00000000000001421 ) ) ;
#10140=CARTESIAN_POINT ( 'NONE',  ( 25.00000000000000000, 0.000000000000000000, 75.00000000000000000 ) ) ;
#10141=CIRCLE ( 'NONE', #21250, 16.23205080756887853 ) ;
#10146=VERTEX_POINT ( 'NONE', #15227 ) ;
#10175=AXIS2_PLACEMENT_3D ( 'NONE', #13372, #5332, #15184 ) ;
#10216=DIRECTION ( 'NONE',  ( -1.000000000000000000, 1.224646799147352714E-16, 0.000000000000000000 ) ) ;
#10235=ORIENTED_EDGE ( 'NONE', *, *, #13403, .F. ) ;
#10247=( GEOMETRIC_REPRESENTATION_CONTEXT ( 3 ) GLOBAL_UNCERTAINTY_ASSIGNED_CONTEXT ( ( #18429 ) ) GLOBAL_UNIT_ASSIGNED_CONTEXT ( ( #3111, #12945, #11257 ) ) REPRESENTATION_CONTEXT ( 'NONE', 'WORKASPACE' ) );
#10248=DIRECTION ( 'NONE',  ( 1.000000000000000000, 0.000000000000000000, -0.000000000000000000 ) ) ;
#10326=PRODUCT ( '360-Degree Detachable Power Base', '360-Degree Detachable Power Base', '', ( #17963 ) ) ;
#10329=DIRECTION ( 'NONE',  ( -0.000000000000000000, -0.000000000000000000, -1.000000000000000000 ) ) ;
#10382=CIRCLE ( 'NONE', #16132, 25.00000000000000000 ) ;
#10407=EDGE_LOOP ( 'NONE', ( #4657, #6829 ) ) ;
#10410=CARTESIAN_POINT ( 'NONE',  ( 22.56777165119825668, 0.000000000000000000, 93.00000000000000000 ) ) ;
#10449=ORIENTED_EDGE ( 'NONE', *, *, #21201, .F. ) ;
#10454=CARTESIAN_POINT ( 'NONE',  ( 0.000000000000000000, 0.000000000000000000, 77.51594804401857175 ) ) ;
#10462=CARTESIAN_POINT ( 'NONE',  ( -10.76782065184847781, 0.1824719560092695203, 91.99999999999998579 ) ) ;
#10479=CARTESIAN_POINT ( 'NONE',  ( -24.63401512838761320, 3.016796777712736283E-15, 77.51594804401857175 ) ) ;
#10529=TOROIDAL_SURFACE ( 'NONE', #12704, 10.76794919243112325, 2.000000000000000000 ) ;
#10549=DIRECTION ( 'NONE',  ( -1.000000000000000000, 0.000000000000000000, 0.000000000000000000 ) ) ;
#10553=DIRECTION ( 'NONE',  ( 0.000000000000000000, 0.000000000000000000, 1.000000000000000000 ) ) ;
#10588=VERTEX_POINT ( 'NONE', #12171 ) ;
#10628=VERTEX_POINT ( 'NONE', #15781 ) ;
#10631=EDGE_LOOP ( 'NONE', ( #16958, #7259 ) ) ;
#10656=DIRECTION ( 'NONE',  ( 0.000000000000000000, 0.000000000000000000, 1.000000000000000000 ) ) ;
#10702=ORIENTED_EDGE ( 'NONE', *, *, #21236, .T. ) ;
#10711=FACE_OUTER_BOUND ( 'NONE', #15390, .T. ) ;
#10736=CIRCLE ( 'NONE', #2452, 2.000000000000001776 ) ;
#10763=DIRECTION ( 'NONE',  ( 0.000000000000000000, 0.000000000000000000, 1.000000000000000000 ) ) ;
#10797=ADVANCED_FACE ( 'NONE', ( #10711 ), #13063, .F. ) ;
#10800=CARTESIAN_POINT ( 'NONE',  ( 24.63401512838761320, 0.000000000000000000, 77.51594804401857175 ) ) ;
#10806=EDGE_LOOP ( 'NONE', ( #2068, #8576 ) ) ;
#10846=AXIS2_PLACEMENT_3D ( 'NONE', #6011, #16373, #20062 ) ;
#10893=DIRECTION ( 'NONE',  ( 0.000000000000000000, 0.000000000000000000, -1.000000000000000000 ) ) ;
#10900=CONICAL_SURFACE ( 'NONE', #3688, 25.00000000000000000, 0.1745329251994333364 ) ;
#10949=CARTESIAN_POINT ( 'NONE',  ( 0.000000000000000000, 0.000000000000000000, 90.00000000000000000 ) ) ;
#10956=ORIENTED_EDGE ( 'NONE', *, *, #4003, .T. ) ;
#10960=VERTEX_POINT ( 'NONE', #17466 ) ;
#10985=AXIS2_PLACEMENT_3D ( 'NONE', #21410, #6108, #825 ) ;
#10993=FACE_BOUND ( 'NONE', #10407, .T. ) ;
#10994=PLANE ( 'NONE',  #11649 ) ;
#11041=CARTESIAN_POINT ( 'NONE',  ( 14.50000000000000178, -3.976862775871337963, 93.00000000000001421 ) ) ;
#11061=FACE_OUTER_BOUND ( 'NONE', #4170, .T. ) ;
#11090=ORIENTED_EDGE ( 'NONE', *, *, #16135, .F. ) ;
#11094=VECTOR ( 'NONE', #12557, 1000.000000000000000 ) ;
#11101=DIRECTION ( 'NONE',  ( 1.000000000000000000, 0.000000000000000000, -0.000000000000000000 ) ) ;
#11147=CARTESIAN_POINT ( 'NONE',  ( 8.999942255032404859, -11.40691176929436068, 93.00000000000000000 ) ) ;
#11225=VERTEX_POINT ( 'NONE', #8192 ) ;
#11234=DIRECTION ( 'NONE',  ( 1.000000000000000000, 0.000000000000000000, 0.000000000000000000 ) ) ;
#11257=( NAMED_UNIT ( * ) SI_UNIT ( $, .STERADIAN. ) SOLID_ANGLE_UNIT ( ) );
#11337=AXIS2_PLACEMENT_3D ( 'NONE', #15980, #2128, #2018 ) ;
#11364=CARTESIAN_POINT ( 'NONE',  ( 13.96913104090061886, 4.808762379633894746, 93.00000000000002842 ) ) ;
#11425=EDGE_LOOP ( 'NONE', ( #19427, #18134 ) ) ;
#11470=CARTESIAN_POINT ( 'NONE',  ( -2.025093002184608082, 14.49031849020018647, 93.00000000000000000 ) ) ;
#11523=CARTESIAN_POINT ( 'NONE',  ( 0.000000000000000000, 0.000000000000000000, 92.00000000000000000 ) ) ;
#11567=AXIS2_PLACEMENT_3D ( 'NONE', #14471, #5902, #6233 ) ;
#11577=CARTESIAN_POINT ( 'NONE',  ( 7.157650466794455824, -8.055668064929562888, 92.00000000000001421 ) ) ;
#11590=CARTESIAN_POINT ( 'NONE',  ( 0.1824719560092671056, 10.76782065184847959, 92.00000000000001421 ) ) ;
#11609=DIRECTION ( 'NONE',  ( 0.000000000000000000, 0.000000000000000000, 1.000000000000000000 ) ) ;
#11620=EDGE_CURVE ( 'NONE', #846, #10588, #3806, .T. ) ;
#11633=AXIS2_PLACEMENT_3D ( 'NONE', #19314, #2425, #11101 ) ;
#11649=AXIS2_PLACEMENT_3D ( 'NONE', #527, #17863, #14599 ) ;
#11674=SURFACE_SIDE_STYLE ('',( #20202 ) ) ;
#11697=CARTESIAN_POINT ( 'NONE',  ( 3.593890535426114141, -10.35670734540880922, 92.00000000000000000 ) ) ;
#11704=AXIS2_PLACEMENT_3D ( 'NONE', #6334, #16693, #14574 ) ;
#11734=AXIS2_PLACEMENT_3D ( 'NONE', #9693, #21491, #14549 ) ;
#11737=ORIENTED_EDGE ( 'NONE', *, *, #16835, .T. ) ;
#11810=CARTESIAN_POINT ( 'NONE',  ( -8.469031667849373335, -6.688043756404093543, 91.99999999999997158 ) ) ;
#11820=CARTESIAN_POINT ( 'NONE',  ( -7.549707216296317469, 7.678935899902893603, 91.99999999999998579 ) ) ;
#11824=DIRECTION ( 'NONE',  ( -0.000000000000000000, -0.000000000000000000, -1.000000000000000000 ) ) ;
#11846=EDGE_LOOP ( 'NONE', ( #19962, #7192 ) ) ;
#11889=CARTESIAN_POINT ( 'NONE',  ( 24.63401512838761320, 0.000000000000000000, 77.51594804401857175 ) ) ;
#11897=( NAMED_UNIT ( * ) PLANE_ANGLE_UNIT ( ) SI_UNIT ( $, .RADIAN. ) );
#11918=CARTESIAN_POINT ( 'NONE',  ( -0.04718088033475312248, -10.76825293233556202, 92.00000000000000000 ) ) ;
#11928=CARTESIAN_POINT ( 'NONE',  ( 2.476137110235832939, 10.55034688490274242, 92.00000000000001421 ) ) ;
#11930=DIRECTION ( 'NONE',  ( 0.000000000000000000, 0.000000000000000000, 1.000000000000000000 ) ) ;
#11985=( NAMED_UNIT ( * ) PLANE_ANGLE_UNIT ( ) SI_UNIT ( $, .RADIAN. ) );
#12032=CARTESIAN_POINT ( 'NONE',  ( -10.75822951548915185, -1.509788170712045297, 92.00000000000002842 ) ) ;
#12033=ORIENTED_EDGE ( 'NONE', *, *, #7496, .F. ) ;
#12099=FILL_AREA_STYLE_COLOUR ( '', #12749 ) ;
#12115=ORIENTED_EDGE ( 'NONE', *, *, #21236, .F. ) ;
#12171=CARTESIAN_POINT ( 'NONE',  ( -10.76794919243112325, 1.318693451189210089E-15, 92.50000000000000000 ) ) ;
#12216=EDGE_CURVE ( 'NONE', #7787, #10628, #5942, .T. ) ;
#12254=VERTEX_POINT ( 'NONE', #19663 ) ;
#12265=CARTESIAN_POINT ( 'NONE',  ( 0.000000000000000000, 0.000000000000000000, 93.00000000000000000 ) ) ;
#12308=AXIS2_PLACEMENT_3D ( 'NONE', #12265, #12383, #17560 ) ;
#12329=CIRCLE ( 'NONE', #15555, 2.000000000000001776 ) ;
#12356=DIRECTION ( 'NONE',  ( -0.000000000000000000, -0.000000000000000000, -1.000000000000000000 ) ) ;
#12378=CARTESIAN_POINT ( 'NONE',  ( -7.580942749559346439, 7.647666590413454202, 92.00000000000000000 ) ) ;
#12383=DIRECTION ( 'NONE',  ( 0.000000000000000000, 0.000000000000000000, 1.000000000000000000 ) ) ;
#12397=DIRECTION ( 'NONE',  ( 0.000000000000000000, 0.000000000000000000, 1.000000000000000000 ) ) ;
#12399=( GEOMETRIC_REPRESENTATION_CONTEXT ( 3 ) GLOBAL_UNCERTAINTY_ASSIGNED_CONTEXT ( ( #2668 ) ) GLOBAL_UNIT_ASSIGNED_CONTEXT ( ( #5436, #11985, #19173 ) ) REPRESENTATION_CONTEXT ( 'NONE', 'WORKASPACE' ) );
#12440=AXIS2_PLACEMENT_3D ( 'NONE', #9102, #434, #10893 ) ;
#12442=DIRECTION ( 'NONE',  ( 1.000000000000000000, 0.000000000000000000, 0.000000000000000000 ) ) ;
#12449=EDGE_CURVE ( 'NONE', #945, #930, #14884, .T. ) ;
#12452=CARTESIAN_POINT ( 'NONE',  ( 0.000000000000000000, 0.000000000000000000, 77.51594804401857175 ) ) ;
#12479=ORIENTED_EDGE ( 'NONE', *, *, #2633, .T. ) ;
#12485=EDGE_LOOP ( 'NONE', ( #22080, #14503, #11737, #3969 ) ) ;
#12504=ORIENTED_EDGE ( 'NONE', *, *, #20966, .T. ) ;
#12535=CIRCLE ( 'NONE', #3168, 14.50000000000000000 ) ;
#12539=ORIENTED_EDGE ( 'NONE', *, *, #1832, .T. ) ;
#12548=CARTESIAN_POINT ( 'NONE',  ( 0.000000000000000000, 0.000000000000000000, 75.00000000000000000 ) ) ;
#12557=DIRECTION ( 'NONE',  ( 0.1736481776669307198, 0.000000000000000000, 0.9848077530122080203 ) ) ;
#12615=CARTESIAN_POINT ( 'NONE',  ( -6.453512288987201195, -13.27786176931083340, 93.00000000000000000 ) ) ;
#12616=CONICAL_SURFACE ( 'NONE', #2888, 23.03038449397558196, 0.1745329251994333364 ) ;
#12623=ORIENTED_EDGE ( 'NONE', *, *, #20925, .T. ) ;
#12667=VERTEX_POINT ( 'NONE', #15178 ) ;
#12676=ORIENTED_EDGE ( 'NONE', *, *, #1423, .T. ) ;
#12704=AXIS2_PLACEMENT_3D ( 'NONE', #7873, #4357, #6280 ) ;
#12716=TOROIDAL_SURFACE ( 'NONE', #17025, 24.63401512838761320, 3.000000000000035083 ) ;
#12749=COLOUR_RGB ( '', 0.40784314, 0.44705882, 0.49803922) ;
#12763=AXIS2_PLACEMENT_3D ( 'NONE', #18000, #12929, #19775 ) ;
#12783=AXIS2_PLACEMENT_3D ( 'NONE', #18612, #13659, #17037 ) ;
#12834=CARTESIAN_POINT ( 'NONE',  ( -9.635142796197669668, 10.84906991693322986, 93.00000000000001421 ) ) ;
#12887=AXIS2_PLACEMENT_3D ( 'NONE', #12452, #20759, #19301 ) ;
#12914=CARTESIAN_POINT ( 'NONE',  ( -10.76794919243112325, 0.000000000000000000, 95.00000000000000000 ) ) ;
#12915=ORIENTED_EDGE ( 'NONE', *, *, #4139, .F. ) ;
#12920=CARTESIAN_POINT ( 'NONE',  ( 0.000000000000000000, 0.000000000000000000, 90.00000000000000000 ) ) ;
#12929=DIRECTION ( 'NONE',  ( -0.000000000000000000, -0.000000000000000000, 1.000000000000000000 ) ) ;
#12939=DIRECTION ( 'NONE',  ( 0.000000000000000000, 0.000000000000000000, 1.000000000000000000 ) ) ;
#12944=CARTESIAN_POINT ( 'NONE',  ( 10.16457016735504304, -10.34237653894239983, 93.00000000000000000 ) ) ;
#12945=( NAMED_UNIT ( * ) PLANE_ANGLE_UNIT ( ) SI_UNIT ( $, .RADIAN. ) );
#13039=EDGE_CURVE ( 'NONE', #15441, #5465, #7292, .T. ) ;
#13049=CARTESIAN_POINT ( 'NONE',  ( 3.344898002356376576, 14.20274344593240556, 92.99999999999997158 ) ) ;
#13063=TOROIDAL_SURFACE ( 'NONE', #4776, 22.56777165119825668, 3.000000000000000000 ) ;
#13065=CONICAL_SURFACE ( 'NONE', #15951, 25.00000000000000000, 0.1745329251994333364 ) ;
#13071=DIRECTION ( 'NONE',  ( 1.000000000000000000, 0.000000000000000000, 0.000000000000000000 ) ) ;
#13131=ORIENTED_EDGE ( 'NONE', *, *, #7732, .F. ) ;
#13149=CARTESIAN_POINT ( 'NONE',  ( -23.03038449397558196, 2.820408665368003469E-15, 75.34729635533385306 ) ) ;
#13161=ORIENTED_EDGE ( 'NONE', *, *, #8982, .T. ) ;
#13163=CARTESIAN_POINT ( 'NONE',  ( -11.67815946035152308, 8.814245471595203441, 93.00000000000001421 ) ) ;
#13200=EDGE_LOOP ( 'NONE', ( #8907, #9407 ) ) ;
#13250=PRODUCT_DEFINITION_CONTEXT ( 'detailed design', #14059, 'design' ) ;
#13268=ORIENTED_EDGE ( 'NONE', *, *, #2358, .T. ) ;
#13270=PLANE ( 'NONE',  #91 ) ;
#13351=CARTESIAN_POINT ( 'NONE',  ( 0.000000000000000000, 0.000000000000000000, 94.00000000000000000 ) ) ;
#13372=CARTESIAN_POINT ( 'NONE',  ( 0.000000000000000000, 0.000000000000000000, 75.00000000000000000 ) ) ;
#13392=CARTESIAN_POINT ( 'NONE',  ( -7.387516090585421580, 7.838405800256096789, 92.00000000000001421 ) ) ;
#13400=CIRCLE ( 'NONE', #5494, 21.63401512838757768 ) ;
#13403=EDGE_CURVE ( 'NONE', #12667, #21337, #21341, .T. ) ;
#13410=ADVANCED_FACE ( 'NONE', ( #18189, #4000 ), #10994, .F. ) ;
#13412=ADVANCED_FACE ( 'NONE', ( #21434 ), #4093, .T. ) ;
#13473=TOROIDAL_SURFACE ( 'NONE', #19217, 22.56777165119825668, 5.000000000000000000 ) ;
#13518=CARTESIAN_POINT ( 'NONE',  ( 0.000000000000000000, 0.000000000000000000, 80.43141006107198621 ) ) ;
#13550=PRODUCT_DEFINITION_FORMATION_WITH_SPECIFIED_SOURCE ( 'ANY', '', #10326, .NOT_KNOWN. ) ;
#13560=CARTESIAN_POINT ( 'NONE',  ( 22.97235139684061878, 0.000000000000000000, 75.01817430661621700 ) ) ;
#13638=ORIENTED_EDGE ( 'NONE', *, *, #7496, .T. ) ;
#13640=ORIENTED_EDGE ( 'NONE', *, *, #14385, .T. ) ;
#13659=DIRECTION ( 'NONE',  ( 1.224646799147353207E-16, 1.000000000000000000, -0.000000000000000000 ) ) ;
#13688=ORIENTED_EDGE ( 'NONE', *, *, #20520, .T. ) ;
#13724=CARTESIAN_POINT ( 'NONE',  ( -10.76794919243112325, 1.318693451189210089E-15, 92.00000000000000000 ) ) ;
#13732=EDGE_CURVE ( 'NONE', #6741, #237, #19548, .T. ) ;
#13763=ORIENTED_EDGE ( 'NONE', *, *, #20966, .F. ) ;
#13810=DIRECTION ( 'NONE',  ( 0.000000000000000000, 0.000000000000000000, 1.000000000000000000 ) ) ;
#13818=AXIS2_PLACEMENT_3D ( 'NONE', #5830, #9663, #19882 ) ;
#13843=CARTESIAN_POINT ( 'NONE',  ( -0.09137847850202075739, -10.76827681573429807, 92.00000000000000000 ) ) ;
#13948=EDGE_LOOP ( 'NONE', ( #5955, #3348, #15235, #4380 ) ) ;
#13953=CARTESIAN_POINT ( 'NONE',  ( -22.56777165119825668, 2.944661181028116692E-15, 93.00000000000000000 ) ) ;
#13961=CARTESIAN_POINT ( 'NONE',  ( -10.76825293233556025, 0.04718088033475291432, 91.99999999999998579 ) ) ;
#13965=PLANE ( 'NONE',  #12308 ) ;
#14032=DIRECTION ( 'NONE',  ( -1.000000000000000000, 1.224646799147351482E-16, 0.000000000000000000 ) ) ;
#14046=PLANE ( 'NONE',  #11633 ) ;
#14051=DIRECTION ( 'NONE',  ( 1.000000000000000000, 0.000000000000000000, 0.000000000000000000 ) ) ;
#14054=LINE ( 'NONE', #10140, #1307 ) ;
#14059=APPLICATION_CONTEXT ( 'automotive_design' ) ;
#14095=VECTOR ( 'NONE', #18126, 1000.000000000000000 ) ;
#14137=CARTESIAN_POINT ( 'NONE',  ( -10.76794919243112325, 0.000000000000000000, 93.00000000000000000 ) ) ;
#14209=AXIS2_PLACEMENT_3D ( 'NONE', #1245, #5883, #4194 ) ;
#14295=MANIFOLD_SOLID_BREP ( 'Revolve1', #17930 ) ;
#14316=CARTESIAN_POINT ( 'NONE',  ( -11.40691176929435535, -8.999942255032468807, 93.00000000000000000 ) ) ;
#14323=VERTEX_POINT ( 'NONE', #10410 ) ;
#14337=FACE_OUTER_BOUND ( 'NONE', #15543, .T. ) ;
#14357=DIRECTION ( 'NONE',  ( 0.1736481776669307198, 0.000000000000000000, 0.9848077530122080203 ) ) ;
#14385=EDGE_CURVE ( 'NONE', #17378, #20879, #6267, .T. ) ;
#14422=CARTESIAN_POINT ( 'NONE',  ( 9.901812489146273322, -10.59772277891044290, 93.00000000000000000 ) ) ;
#14453=DIRECTION ( 'NONE',  ( 0.000000000000000000, 0.000000000000000000, 1.000000000000000000 ) ) ;
#14465=EDGE_LOOP ( 'NONE', ( #6477, #3465, #6397, #20070 ) ) ;
#14471=CARTESIAN_POINT ( 'NONE',  ( 0.000000000000000000, 0.000000000000000000, 75.00000000000000000 ) ) ;
#14503=ORIENTED_EDGE ( 'NONE', *, *, #13039, .T. ) ;
#14511=CIRCLE ( 'NONE', #8043, 5.000000000000000888 ) ;
#14531=FACE_BOUND ( 'NONE', #13200, .T. ) ;
#14549=DIRECTION ( 'NONE',  ( -1.000000000000000000, 1.224646799147353454E-16, 0.000000000000000000 ) ) ;
#14574=DIRECTION ( 'NONE',  ( 1.000000000000000000, 0.000000000000000000, 0.000000000000000000 ) ) ;
#14599=DIRECTION ( 'NONE',  ( 1.000000000000000000, 0.000000000000000000, -0.000000000000000000 ) ) ;
#14617=ORIENTED_EDGE ( 'NONE', *, *, #3361, .T. ) ;
#14623=CIRCLE ( 'NONE', #7071, 22.56777165119825668 ) ;
#14696=TOROIDAL_SURFACE ( 'NONE', #12887, 24.63401512838761320, 3.000000000000035083 ) ;
#14716=ORIENTED_EDGE ( 'NONE', *, *, #13732, .F. ) ;
#14749=CARTESIAN_POINT ( 'NONE',  ( -0.8583760989383530937, -14.48452571672253697, 93.00000000000001421 ) ) ;
#14769=CONICAL_SURFACE ( 'NONE', #8706, 23.03038449397558196, 0.1745329251994333364 ) ;
#14804=CIRCLE ( 'NONE', #11567, 22.96914677622851642 ) ;
#14862=ADVANCED_FACE ( 'NONE', ( #4084 ), #13473, .T. ) ;
#14884=CIRCLE ( 'NONE', #13818, 22.97235139684061878 ) ;
#14918=DIRECTION ( 'NONE',  ( 0.000000000000000000, 0.000000000000000000, 1.000000000000000000 ) ) ;
#14944=DIRECTION ( 'NONE',  ( 0.000000000000000000, 0.000000000000000000, -1.000000000000000000 ) ) ;
#14947=CIRCLE ( 'NONE', #12783, 2.999999999999999112 ) ;
#14977=AXIS2_PLACEMENT_3D ( 'NONE', #2705, #9589, #1024 ) ;
#15033=ORIENTED_EDGE ( 'NONE', *, *, #627, .F. ) ;
#15085=CARTESIAN_POINT ( 'NONE',  ( -14.50030254718125100, 0.06328415631827216670, 93.00000000000005684 ) ) ;
#15097=CARTESIAN_POINT ( 'NONE',  ( 14.50000000000000000, 0.000000000000000000, 92.50000000000000000 ) ) ;
#15166=CARTESIAN_POINT ( 'NONE',  ( -27.49181041625929467, 3.366775762903781044E-15, 89.13175911166534604 ) ) ;
#15178=CARTESIAN_POINT ( 'NONE',  ( 16.23205080756887853, 0.000000000000000000, 95.00000000000000000 ) ) ;
#15184=DIRECTION ( 'NONE',  ( 1.000000000000000000, 0.000000000000000000, 0.000000000000000000 ) ) ;
#15194=CARTESIAN_POINT ( 'NONE',  ( -9.211115167980509000, -5.709328484389684100, 92.00000000000001421 ) ) ;
#15208=PLANE ( 'NONE',  #88 ) ;
#15223=VERTEX_POINT ( 'NONE', #115 ) ;
#15227=CARTESIAN_POINT ( 'NONE',  ( 22.96914677622851642, 0.000000000000000000, 75.00000000000000000 ) ) ;
#15235=ORIENTED_EDGE ( 'NONE', *, *, #7732, .T. ) ;
#15334=ORIENTED_EDGE ( 'NONE', *, *, #15829, .T. ) ;
#15390=EDGE_LOOP ( 'NONE', ( #1514, #7272, #6137, #13763 ) ) ;
#15418=CARTESIAN_POINT ( 'NONE',  ( -14.50024104873820185, 0.1235481402557507408, 93.00000000000000000 ) ) ;
#15427=CARTESIAN_POINT ( 'NONE',  ( 1.259348629394230867, 10.71767081544559552, 92.00000000000001421 ) ) ;
#15441=VERTEX_POINT ( 'NONE', #20465 ) ;
#15495=DIRECTION ( 'NONE',  ( -0.000000000000000000, -0.000000000000000000, -1.000000000000000000 ) ) ;
#15503=DIRECTION ( 'NONE',  ( -0.000000000000000000, -0.000000000000000000, 1.000000000000000000 ) ) ;
#15518=CARTESIAN_POINT ( 'NONE',  ( -0.3188271712753658615, -10.76635261883074435, 92.00000000000002842 ) ) ;
#15529=CARTESIAN_POINT ( 'NONE',  ( 0.09137847850201968880, 10.76827681573430517, 92.00000000000001421 ) ) ;
#15543=EDGE_LOOP ( 'NONE', ( #12115, #9289, #9326, #2079 ) ) ;
#15546=TOROIDAL_SURFACE ( 'NONE', #9090, 16.23205080756887853, 2.000000000000000000 ) ;
#15555=AXIS2_PLACEMENT_3D ( 'NONE', #16837, #4445, #18196 ) ;
#15699=ORIENTED_EDGE ( 'NONE', *, *, #10065, .F. ) ;
#15734=CARTESIAN_POINT ( 'NONE',  ( -25.00000000000000000, 3.061616997868383043E-15, 75.00000000000000000 ) ) ;
#15773=EDGE_LOOP ( 'NONE', ( #12033, #17829 ) ) ;
#15781=CARTESIAN_POINT ( 'NONE',  ( -25.52219491023488018, 3.125567430403401865E-15, 89.47905546699919910 ) ) ;
#15811=ORIENTED_EDGE ( 'NONE', *, *, #11620, .T. ) ;
#15829=EDGE_CURVE ( 'NONE', #15223, #6741, #1982, .T. ) ;
#15879=ORIENTED_EDGE ( 'NONE', *, *, #7546, .F. ) ;
#15951=AXIS2_PLACEMENT_3D ( 'NONE', #19318, #10553, #14051 ) ;
#15957=EDGE_CURVE ( 'NONE', #20136, #2853, #22107, .T. ) ;
#15980=CARTESIAN_POINT ( 'NONE',  ( 0.000000000000000000, 0.000000000000000000, 95.00000000000000000 ) ) ;
#16020=DIRECTION ( 'NONE',  ( 1.000000000000000000, 0.000000000000000000, 0.000000000000000000 ) ) ;
#16030=EDGE_LOOP ( 'NONE', ( #11090, #7413, #7481, #4790 ) ) ;
#16107=CARTESIAN_POINT ( 'NONE',  ( -10.55583158923998077, -9.946257437971063098, 93.00000000000002842 ) ) ;
#16132=AXIS2_PLACEMENT_3D ( 'NONE', #217, #17436, #7086 ) ;
#16135=EDGE_CURVE ( 'NONE', #7787, #15223, #192, .T. ) ;
#16145=DIRECTION ( 'NONE',  ( 0.000000000000000000, -1.000000000000000000, 0.000000000000000000 ) ) ;
#16173=CARTESIAN_POINT ( 'NONE',  ( 21.63401512838757768, 0.000000000000000000, 77.51594804401857175 ) ) ;
#16208=CARTESIAN_POINT ( 'NONE',  ( 8.814245471595175019, 11.67815946035151953, 93.00000000000000000 ) ) ;
#16226=DIRECTION ( 'NONE',  ( 0.000000000000000000, 0.000000000000000000, 1.000000000000000000 ) ) ;
#16250=FACE_OUTER_BOUND ( 'NONE', #12485, .T. ) ;
#16319=CARTESIAN_POINT ( 'NONE',  ( 0.1235481402557489783, 14.50024104873819830, 92.99999999999998579 ) ) ;
#16361=AXIS2_PLACEMENT_3D ( 'NONE', #506, #16145, #7382 ) ;
#16373=DIRECTION ( 'NONE',  ( 0.000000000000000000, 0.000000000000000000, 1.000000000000000000 ) ) ;
#16382=EDGE_LOOP ( 'NONE', ( #5216, #21843, #12504, #13638 ) ) ;
#16411=DIRECTION ( 'NONE',  ( 0.000000000000000000, 0.000000000000000000, 1.000000000000000000 ) ) ;
#16413=CIRCLE ( 'NONE', #3822, 14.50000000000000000 ) ;
#16446=EDGE_LOOP ( 'NONE', ( #3633, #5077, #2000, #15334 ) ) ;
#16535=CARTESIAN_POINT ( 'NONE',  ( -10.07820250684337537, 10.42709000561872479, 92.99999999999998579 ) ) ;
#16572=VERTEX_POINT ( 'NONE', #16865 ) ;
#16647=CARTESIAN_POINT ( 'NONE',  ( 14.50000000000000000, 0.000000000000000000, 93.00000000000000000 ) ) ;
#16669=ADVANCED_FACE ( 'NONE', ( #8983 ), #13065, .T. ) ;
#16678=PLANE ( 'NONE',  #9818 ) ;
#16693=DIRECTION ( 'NONE',  ( 0.000000000000000000, 0.000000000000000000, 1.000000000000000000 ) ) ;
#16763=CARTESIAN_POINT ( 'NONE',  ( -14.50000000000000000, 1.775737858763662015E-15, 93.00000000000000000 ) ) ;
#16770=AXIS2_PLACEMENT_3D ( 'NONE', #13518, #4951, #5059 ) ;
#16776=CARTESIAN_POINT ( 'NONE',  ( -5.709328484389660119, 9.211115167980505447, 92.00000000000000000 ) ) ;
#16816=CARTESIAN_POINT ( 'NONE',  ( 25.52219491023488018, 0.000000000000000000, 89.47905546699919910 ) ) ;
#16835=EDGE_CURVE ( 'NONE', #5465, #20525, #133, .T. ) ;
#16837=CARTESIAN_POINT ( 'NONE',  ( 16.23205080756887853, 0.000000000000000000, 93.00000000000000000 ) ) ;
#16850=CARTESIAN_POINT ( 'NONE',  ( 0.000000000000000000, 0.000000000000000000, 95.00000000000000000 ) ) ;
#16859=FACE_OUTER_BOUND ( 'NONE', #14465, .T. ) ;
#16865=CARTESIAN_POINT ( 'NONE',  ( -14.50000000000000000, 1.881795382636152632E-15, 94.00000000000000000 ) ) ;
#16877=EDGE_LOOP ( 'NONE', ( #3322, #3889, #13688, #6020 ) ) ;
#16889=ADVANCED_FACE ( 'NONE', ( #16859 ), #1209, .F. ) ;
#16958=ORIENTED_EDGE ( 'NONE', *, *, #21201, .T. ) ;
#16987=CARTESIAN_POINT ( 'NONE',  ( -4.782033626261148029, -9.864562363145054746, 92.00000000000000000 ) ) ;
#17008=DIRECTION ( 'NONE',  ( 0.1736481776669307198, 0.000000000000000000, 0.9848077530122080203 ) ) ;
#17023=CIRCLE ( 'NONE', #1188, 27.49181041625929112 ) ;
#17025=AXIS2_PLACEMENT_3D ( 'NONE', #18662, #15503, #7067 ) ;
#17037=DIRECTION ( 'NONE',  ( -1.000000000000000000, 1.224646799147353454E-16, 0.000000000000000000 ) ) ;
#17080=( NAMED_UNIT ( * ) SI_UNIT ( $, .STERADIAN. ) SOLID_ANGLE_UNIT ( ) );
#17108=ADVANCED_FACE ( 'NONE', ( #8642 ), #12716, .T. ) ;
#17139=ORIENTED_EDGE ( 'NONE', *, *, #20686, .T. ) ;
#17175=ORIENTED_EDGE ( 'NONE', *, *, #8982, .F. ) ;
#17208=CARTESIAN_POINT ( 'NONE',  ( -1.259348629394223984, -10.71767081544559375, 91.99999999999998579 ) ) ;
#17298=CARTESIAN_POINT ( 'NONE',  ( -22.56777165119825668, 2.763754931652832307E-15, 90.00000000000000000 ) ) ;
#17310=ADVANCED_FACE ( 'NONE', ( #22022 ), #2274, .T. ) ;
#17325=CARTESIAN_POINT ( 'NONE',  ( -10.71767081544559908, 1.259348629394239083, 92.00000000000002842 ) ) ;
#17329=FACE_OUTER_BOUND ( 'NONE', #8948, .T. ) ;
#17378=VERTEX_POINT ( 'NONE', #18981 ) ;
#17436=DIRECTION ( 'NONE',  ( 0.000000000000000000, 0.000000000000000000, 1.000000000000000000 ) ) ;
#17443=PRODUCT_DEFINITION ( 'UNKNOWN', '', #13550, #13250 ) ;
#17464=FACE_OUTER_BOUND ( 'NONE', #7987, .T. ) ;
#17466=CARTESIAN_POINT ( 'NONE',  ( -14.50000000000000000, 1.775737858763662015E-15, 92.50000000000000000 ) ) ;
#17488=DIRECTION ( 'NONE',  ( 0.000000000000000000, 0.000000000000000000, 1.000000000000000000 ) ) ;
#17508=CARTESIAN_POINT ( 'NONE',  ( 12.50000000000000000, 1.530808498934191521E-15, 94.00000000000000000 ) ) ;
#17519=EDGE_CURVE ( 'NONE', #5465, #2853, #14511, .T. ) ;
#17559=DIRECTION ( 'NONE',  ( 0.000000000000000000, -1.000000000000000000, 0.000000000000000000 ) ) ;
#17560=DIRECTION ( 'NONE',  ( 1.000000000000000000, 0.000000000000000000, -0.000000000000000000 ) ) ;
#17596=CARTESIAN_POINT ( 'NONE',  ( 0.000000000000000000, 0.000000000000000000, 75.34729635533385306 ) ) ;
#17628=DIRECTION ( 'NONE',  ( 1.000000000000000000, 0.000000000000000000, 0.000000000000000000 ) ) ;
#17655=EDGE_LOOP ( 'NONE', ( #15811, #298 ) ) ;
#17662=CARTESIAN_POINT ( 'NONE',  ( -9.864562363145052970, 4.782033626261182668, 92.00000000000000000 ) ) ;
#17726=CARTESIAN_POINT ( 'NONE',  ( 27.49181041625929467, 0.000000000000000000, 89.13175911166534604 ) ) ;
#17738=DIRECTION ( 'NONE',  ( 1.224646799147353207E-16, 1.000000000000000000, -0.000000000000000000 ) ) ;
#17753=DIRECTION ( 'NONE',  ( -0.000000000000000000, -0.000000000000000000, 1.000000000000000000 ) ) ;
#17779=CARTESIAN_POINT ( 'NONE',  ( -10.76635261883074435, 0.3188271712753679710, 92.00000000000002842 ) ) ;
#17806=EDGE_LOOP ( 'NONE', ( #1758, #3931, #8289, #9219 ) ) ;
#17819=AXIS2_PLACEMENT_3D ( 'NONE', #10800, #17559, #2236 ) ;
#17829=ORIENTED_EDGE ( 'NONE', *, *, #7781, .F. ) ;
#17862=FACE_OUTER_BOUND ( 'NONE', #11846, .T. ) ;
#17863=DIRECTION ( 'NONE',  ( 0.000000000000000000, 0.000000000000000000, 1.000000000000000000 ) ) ;
#17880=CARTESIAN_POINT ( 'NONE',  ( -22.56777165119825668, 3.065265347278306676E-15, 95.00000000000000000 ) ) ;
#17902=CARTESIAN_POINT ( 'NONE',  ( 14.49999999999999645, 2.015503622133300698, 92.99999999999998579 ) ) ;
#17930=CLOSED_SHELL ( 'NONE', ( #13412, #2192, #5939, #10797, #4169, #17310, #1311, #14862, #20693, #9600, #16889, #16669, #18065, #18766, #9300, #1686, #9735, #19033, #19818, #17108, #19225, #751, #13410, #5698, #6230 ) ) ;
#17963=PRODUCT_CONTEXT ( 'NONE', #19060, 'mechanical' ) ;
#17996=DIRECTION ( 'NONE',  ( -0.1736481776669307198, 2.126576849575776229E-17, 0.9848077530122080203 ) ) ;
#18000=CARTESIAN_POINT ( 'NONE',  ( 0.000000000000000000, 0.000000000000000000, 80.43141006107198621 ) ) ;
#18010=FACE_OUTER_BOUND ( 'NONE', #11425, .T. ) ;
#18015=CARTESIAN_POINT ( 'NONE',  ( -23.03038449397558196, 2.820408665368003469E-15, 75.34729635533385306 ) ) ;
#18028=CARTESIAN_POINT ( 'NONE',  ( 0.000000000000000000, 0.000000000000000000, 0.000000000000000000 ) ) ;
#18061=FACE_OUTER_BOUND ( 'NONE', #10806, .T. ) ;
#18065=ADVANCED_FACE ( 'NONE', ( #10993, #17862 ), #14046, .T. ) ;
#18111=B_SPLINE_CURVE_WITH_KNOTS ( 'NONE', 3,
 ( #4269, #2693, #7554, #19460, #14316, #7887, #16107, #4372, #19789, #21255, #21478, #12615, #5736, #680, #14749, #21590, #5847, #19903, #4049, #9464, #7448, #9247, #11147, #9575, #14422, #6179, #12944, #1012, #11041, #4160 ),
 .UNSPECIFIED., .F., .F.,
 ( 4, 1, 1, 1, 1, 1, 2, 2, 1, 1, 1, 1, 1, 2, 2, 1, 1, 1, 1, 2, 2, 4 ),
 ( 0.5000000000000000000, 0.5624999999999992228, 0.5937499999999988898, 0.6093749999999986677, 0.6171874999999985567, 0.6210937499999984457, 0.6230468749999984457, 0.6249999999999984457, 0.6874999999999985567, 0.7187499999999985567, 0.7343749999999986677, 0.7421874999999986677, 0.7460937499999986677, 0.7480468749999986677, 0.7499999999999986677, 0.8124999999999988898, 0.8437499999999988898, 0.8593749999999988898, 0.8671874999999988898, 0.8710937499999988898, 0.8749999999999988898, 1.000000000000000000 ),
 .UNSPECIFIED. ) ;
#18121=CARTESIAN_POINT ( 'NONE',  ( 0.000000000000000000, 0.000000000000000000, 94.00000000000000000 ) ) ;
#18126=DIRECTION ( 'NONE',  ( -0.1736481776669307198, 2.126576849575776229E-17, 0.9848077530122080203 ) ) ;
#18134=ORIENTED_EDGE ( 'NONE', *, *, #7546, .T. ) ;
#18149=MECHANICAL_DESIGN_GEOMETRIC_PRESENTATION_REPRESENTATION('',(#18518),#7020);
#18176=CARTESIAN_POINT ( 'NONE',  ( 14.50000000000000000, 0.000000000000000000, 94.00000000000000000 ) ) ;
#18189=FACE_BOUND ( 'NONE', #1976, .T. ) ;
#18196=DIRECTION ( 'NONE',  ( 0.000000000000000000, 0.000000000000000000, -1.000000000000000000 ) ) ;
#18233=CARTESIAN_POINT ( 'NONE',  ( -8.999942255032427951, 11.40691176929435535, 93.00000000000001421 ) ) ;
#18252=CARTESIAN_POINT ( 'NONE',  ( 0.000000000000000000, 0.000000000000000000, 94.00000000000000000 ) ) ;
#18324=DIRECTION ( 'NONE',  ( 0.000000000000000000, 0.000000000000000000, 1.000000000000000000 ) ) ;
#18422=DIRECTION ( 'NONE',  ( 0.000000000000000000, 0.000000000000000000, 1.000000000000000000 ) ) ;
#18429=UNCERTAINTY_MEASURE_WITH_UNIT (LENGTH_MEASURE( 1.000000000000000082E-05 ), #3111, 'distance_accuracy_value', 'NONE');
#18462=CARTESIAN_POINT ( 'NONE',  ( -1.509788170712026423, 10.75822951548914830, 91.99999999999998579 ) ) ;
#18518=STYLED_ITEM ( 'NONE', ( #10101 ), #21175 ) ;
#18550=DIRECTION ( 'NONE',  ( 1.000000000000000000, 0.000000000000000000, 0.000000000000000000 ) ) ;
#18566=CARTESIAN_POINT ( 'NONE',  ( 7.548384491377941430, -7.680646770330602280, 91.99999999999998579 ) ) ;
#18578=CARTESIAN_POINT ( 'NONE',  ( 7.871778267153376696, 7.352373015921426891, 92.00000000000000000 ) ) ;
#18612=CARTESIAN_POINT ( 'NONE',  ( -22.56777165119825668, 2.763754931652832307E-15, 90.00000000000000000 ) ) ;
#18642=VERTEX_POINT ( 'NONE', #15097 ) ;
#18662=CARTESIAN_POINT ( 'NONE',  ( 0.000000000000000000, 0.000000000000000000, 77.51594804401857175 ) ) ;
#18677=CARTESIAN_POINT ( 'NONE',  ( -14.20274344593240734, 3.344898002356411659, 93.00000000000000000 ) ) ;
#18690=DIRECTION ( 'NONE',  ( 1.000000000000000000, 0.000000000000000000, 0.000000000000000000 ) ) ;
#18766=ADVANCED_FACE ( 'NONE', ( #20125, #3142 ), #15208, .F. ) ;
#18784=CARTESIAN_POINT ( 'NONE',  ( -7.647666590413455090, -7.580942749559344662, 92.00000000000000000 ) ) ;
#18814=AXIS2_PLACEMENT_3D ( 'NONE', #17596, #2163, #9043 ) ;
#18896=EDGE_CURVE ( 'NONE', #10628, #497, #8364, .T. ) ;
#18954=SURFACE_SIDE_STYLE ('',( #282 ) ) ;
#18981=CARTESIAN_POINT ( 'NONE',  ( 10.76794919243112325, 1.424750975061700904E-15, 95.00000000000000000 ) ) ;
#18999=ORIENTED_EDGE ( 'NONE', *, *, #8253, .T. ) ;
#19008=CARTESIAN_POINT ( 'NONE',  ( -10.55034688490273709, 2.476137110235850258, 92.00000000000001421 ) ) ;
#19033=ADVANCED_FACE ( 'NONE', ( #17329 ), #15546, .T. ) ;
#19057=ORIENTED_EDGE ( 'NONE', *, *, #2080, .F. ) ;
#19060=APPLICATION_CONTEXT ( 'automotive_design' ) ;
#19075=CARTESIAN_POINT ( 'NONE',  ( 23.03038449397558196, 0.000000000000000000, 75.34729635533385306 ) ) ;
#19159=DIRECTION ( 'NONE',  ( 1.000000000000000000, 0.000000000000000000, 0.000000000000000000 ) ) ;
#19173=( NAMED_UNIT ( * ) SI_UNIT ( $, .STERADIAN. ) SOLID_ANGLE_UNIT ( ) );
#19177=VECTOR ( 'NONE', #17996, 1000.000000000000000 ) ;
#19217=AXIS2_PLACEMENT_3D ( 'NONE', #9279, #14453, #2175 ) ;
#19225=ADVANCED_FACE ( 'NONE', ( #20804 ), #13965, .F. ) ;
#19285=ORIENTED_EDGE ( 'NONE', *, *, #1027, .T. ) ;
#19292=DIRECTION ( 'NONE',  ( 0.000000000000000000, -1.000000000000000000, 0.000000000000000000 ) ) ;
#19301=DIRECTION ( 'NONE',  ( 1.000000000000000000, 0.000000000000000000, 0.000000000000000000 ) ) ;
#19305=FACE_OUTER_BOUND ( 'NONE', #16030, .T. ) ;
#19314=CARTESIAN_POINT ( 'NONE',  ( 0.000000000000000000, 0.000000000000000000, 95.00000000000000000 ) ) ;
#19318=CARTESIAN_POINT ( 'NONE',  ( 0.000000000000000000, 0.000000000000000000, 75.00000000000000000 ) ) ;
#19378=DIRECTION ( 'NONE',  ( 0.000000000000000000, 0.000000000000000000, 1.000000000000000000 ) ) ;
#19395=CARTESIAN_POINT ( 'NONE',  ( 23.03038449397558196, 0.000000000000000000, 75.34729635533385306 ) ) ;
#19416=DIRECTION ( 'NONE',  ( -0.000000000000000000, -0.000000000000000000, -1.000000000000000000 ) ) ;
#19427=ORIENTED_EDGE ( 'NONE', *, *, #3630, .T. ) ;
#19460=CARTESIAN_POINT ( 'NONE',  ( -12.40805626191516708, -7.677656142228116209, 93.00000000000000000 ) ) ;
#19462=AXIS2_PLACEMENT_3D ( 'NONE', #10479, #21043, #5518 ) ;
#19502=DIRECTION ( 'NONE',  ( 1.000000000000000000, 0.000000000000000000, 0.000000000000000000 ) ) ;
#19508=CONICAL_SURFACE ( 'NONE', #18814, 23.03038449397558196, 0.1745329251994333364 ) ;
#19548=CIRCLE ( 'NONE', #9855, 21.63401512838757768 ) ;
#19663=CARTESIAN_POINT ( 'NONE',  ( -12.50000000000000000, 0.000000000000000000, 94.00000000000000000 ) ) ;
#19704=FACE_OUTER_BOUND ( 'NONE', #10631, .T. ) ;
#19775=DIRECTION ( 'NONE',  ( 1.000000000000000000, 0.000000000000000000, 0.000000000000000000 ) ) ;
#19789=CARTESIAN_POINT ( 'NONE',  ( -10.34058050218014735, -10.16585704662449174, 93.00000000000000000 ) ) ;
#19818=ADVANCED_FACE ( 'NONE', ( #9667 ), #10529, .T. ) ;
#19882=DIRECTION ( 'NONE',  ( 1.000000000000000000, 0.000000000000000000, 0.000000000000000000 ) ) ;
#19897=CARTESIAN_POINT ( 'NONE',  ( 1.701984465643877398, 14.42982486328545555, 93.00000000000002842 ) ) ;
#19903=CARTESIAN_POINT ( 'NONE',  ( -0.1235481402557490893, -14.50024104873819830, 92.99999999999998579 ) ) ;
#19962=ORIENTED_EDGE ( 'NONE', *, *, #15957, .T. ) ;
#19998=EDGE_CURVE ( 'NONE', #11225, #15441, #5132, .T. ) ;
#20008=CARTESIAN_POINT ( 'NONE',  ( 0.8583760989383623086, 14.48452571672253519, 93.00000000000000000 ) ) ;
#20044=ORIENTED_EDGE ( 'NONE', *, *, #9377, .F. ) ;
#20046=CIRCLE ( 'NONE', #5317, 3.000000000000030198 ) ;
#20062=DIRECTION ( 'NONE',  ( 1.000000000000000000, 0.000000000000000000, 0.000000000000000000 ) ) ;
#20070=ORIENTED_EDGE ( 'NONE', *, *, #12449, .T. ) ;
#20123=CARTESIAN_POINT ( 'NONE',  ( 6.539635590297932843, 8.674798497629369720, 92.00000000000001421 ) ) ;
#20125=FACE_OUTER_BOUND ( 'NONE', #7107, .T. ) ;
#20136=VERTEX_POINT ( 'NONE', #8845 ) ;
#20202=SURFACE_STYLE_FILL_AREA ( #21901 ) ;
#20235=CARTESIAN_POINT ( 'NONE',  ( 7.744474050657649045, 7.483908733559392346, 92.00000000000000000 ) ) ;
#20263=ORIENTED_EDGE ( 'NONE', *, *, #15829, .F. ) ;
#20338=CARTESIAN_POINT ( 'NONE',  ( -2.476137110235820948, -10.55034688490274242, 92.00000000000001421 ) ) ;
#20450=EDGE_LOOP ( 'NONE', ( #15033, #13640, #7962, #7218 ) ) ;
#20465=CARTESIAN_POINT ( 'NONE',  ( -25.00000000000000000, 3.214196380386082240E-15, 75.00000000000000000 ) ) ;
#20520=EDGE_CURVE ( 'NONE', #15223, #497, #20976, .T. ) ;
#20525=VERTEX_POINT ( 'NONE', #17726 ) ;
#20546=CARTESIAN_POINT ( 'NONE',  ( 0.000000000000000000, 0.000000000000000000, 93.00000000000000000 ) ) ;
#20589=EDGE_LOOP ( 'NONE', ( #13131, #17139, #14617, #20044 ) ) ;
#20633=MECHANICAL_DESIGN_GEOMETRIC_PRESENTATION_REPRESENTATION('',(#7000),#12399);
#20675=CIRCLE ( 'NONE', #10985, 10.76794919243112325 ) ;
#20680=CARTESIAN_POINT ( 'NONE',  ( -22.96914677622851642, 2.813105434284154191E-15, 75.00000000000000000 ) ) ;
#20686=EDGE_CURVE ( 'NONE', #237, #6741, #13400, .T. ) ;
#20693=ADVANCED_FACE ( 'NONE', ( #16250 ), #10900, .T. ) ;
#20759=DIRECTION ( 'NONE',  ( -0.000000000000000000, -0.000000000000000000, 1.000000000000000000 ) ) ;
#20779=CIRCLE ( 'NONE', #21498, 12.50000000000000000 ) ;
#20804=FACE_OUTER_BOUND ( 'NONE', #21229, .T. ) ;
#20848=ORIENTED_EDGE ( 'NONE', *, *, #19998, .F. ) ;
#20868=FACE_OUTER_BOUND ( 'NONE', #5101, .T. ) ;
#20879=VERTEX_POINT ( 'NONE', #17508 ) ;
#20898=AXIS2_PLACEMENT_3D ( 'NONE', #2143, #12397, #8913 ) ;
#20925=EDGE_CURVE ( 'NONE', #2791, #12254, #3795, .T. ) ;
#20937=CIRCLE ( 'NONE', #1898, 22.97235139684061878 ) ;
#20966=EDGE_CURVE ( 'NONE', #497, #14323, #6298, .T. ) ;
#20976=LINE ( 'NONE', #19395, #7661 ) ;
#21027=AXIS2_PLACEMENT_3D ( 'NONE', #14137, #19292, #7591 ) ;
#21043=DIRECTION ( 'NONE',  ( 1.224646799147353207E-16, 1.000000000000000000, 0.000000000000000000 ) ) ;
#21175=ADVANCED_BREP_SHAPE_REPRESENTATION ( '', ( #14295, #6677 ), #10247 ) ;
#21194=EDGE_LOOP ( 'NONE', ( #6878, #10449, #12623, #10956 ) ) ;
#21201=EDGE_CURVE ( 'NONE', #2791, #17378, #20675, .T. ) ;
#21204=FACE_OUTER_BOUND ( 'NONE', #16382, .T. ) ;
#21229=EDGE_LOOP ( 'NONE', ( #9, #19057 ) ) ;
#21236=EDGE_CURVE ( 'NONE', #1916, #10146, #21392, .T. ) ;
#21250=AXIS2_PLACEMENT_3D ( 'NONE', #16850, #15495, #22241 ) ;
#21255=CARTESIAN_POINT ( 'NONE',  ( -10.29801091644274713, -10.20851360429410803, 92.99999999999998579 ) ) ;
#21337=VERTEX_POINT ( 'NONE', #2837 ) ;
#21341=CIRCLE ( 'NONE', #2295, 16.23205080756887853 ) ;
#21392=CIRCLE ( 'NONE', #11704, 22.96914677622851642 ) ;
#21410=CARTESIAN_POINT ( 'NONE',  ( 0.000000000000000000, 0.000000000000000000, 95.00000000000000000 ) ) ;
#21434=FACE_OUTER_BOUND ( 'NONE', #20589, .T. ) ;
#21473=CARTESIAN_POINT ( 'NONE',  ( 10.85304084868705843, 9.631209652036005764, 93.00000000000002842 ) ) ;
#21478=CARTESIAN_POINT ( 'NONE',  ( -8.814245471595155479, -11.67815946035151775, 92.99999999999997158 ) ) ;
#21486=ORIENTED_EDGE ( 'NONE', *, *, #17519, .F. ) ;
#21491=DIRECTION ( 'NONE',  ( 1.224646799147353207E-16, 1.000000000000000000, 0.000000000000000000 ) ) ;
#21498=AXIS2_PLACEMENT_3D ( 'NONE', #6940, #13810, #7391 ) ;
#21501=DIRECTION ( 'NONE',  ( -0.000000000000000000, -0.000000000000000000, -1.000000000000000000 ) ) ;
#21557=DIRECTION ( 'NONE',  ( 1.000000000000000000, 0.000000000000000000, 0.000000000000000000 ) ) ;
#21590=CARTESIAN_POINT ( 'NONE',  ( -0.4310340159982842256, -14.49716617963122189, 93.00000000000000000 ) ) ;
#21646=EDGE_CURVE ( 'NONE', #10628, #2661, #14947, .T. ) ;
#21811=CARTESIAN_POINT ( 'NONE',  ( 0.2467007162552592447, 14.49943138577569179, 93.00000000000001421 ) ) ;
#21843=ORIENTED_EDGE ( 'NONE', *, *, #18896, .T. ) ;
#21864=FACE_BOUND ( 'NONE', #17655, .T. ) ;
#21878=CARTESIAN_POINT ( 'NONE',  ( 0.000000000000000000, 0.000000000000000000, 77.51594804401857175 ) ) ;
#21901=FILL_AREA_STYLE ('',( #1322 ) ) ;
#22013=SURFACE_STYLE_USAGE ( .BOTH. , #11674 ) ;
#22022=FACE_OUTER_BOUND ( 'NONE', #20450, .T. ) ;
#22054=CARTESIAN_POINT ( 'NONE',  ( 0.000000000000000000, 0.000000000000000000, 75.00000000000000000 ) ) ;
#22080=ORIENTED_EDGE ( 'NONE', *, *, #19998, .T. ) ;
#22098=CARTESIAN_POINT ( 'NONE',  ( 10.76794919243112325, 0.000000000000000000, 92.50000000000000000 ) ) ;
#22107=CIRCLE ( 'NONE', #11337, 22.56777165119825668 ) ;
#22130=EDGE_LOOP ( 'NONE', ( #3012, #10702 ) ) ;
#22158=CARTESIAN_POINT ( 'NONE',  ( -10.35670734540881277, -3.593890535426112365, 92.00000000000001421 ) ) ;
#22164=CIRCLE ( 'NONE', #11734, 3.000000000000033751 ) ;
#22238=EDGE_LOOP ( 'NONE', ( #5042, #12479, #1180, #5387 ) ) ;
#22241=DIRECTION ( 'NONE',  ( 1.000000000000000000, 0.000000000000000000, 0.000000000000000000 ) ) ;
ENDSEC;
END-ISO-10303-21;
